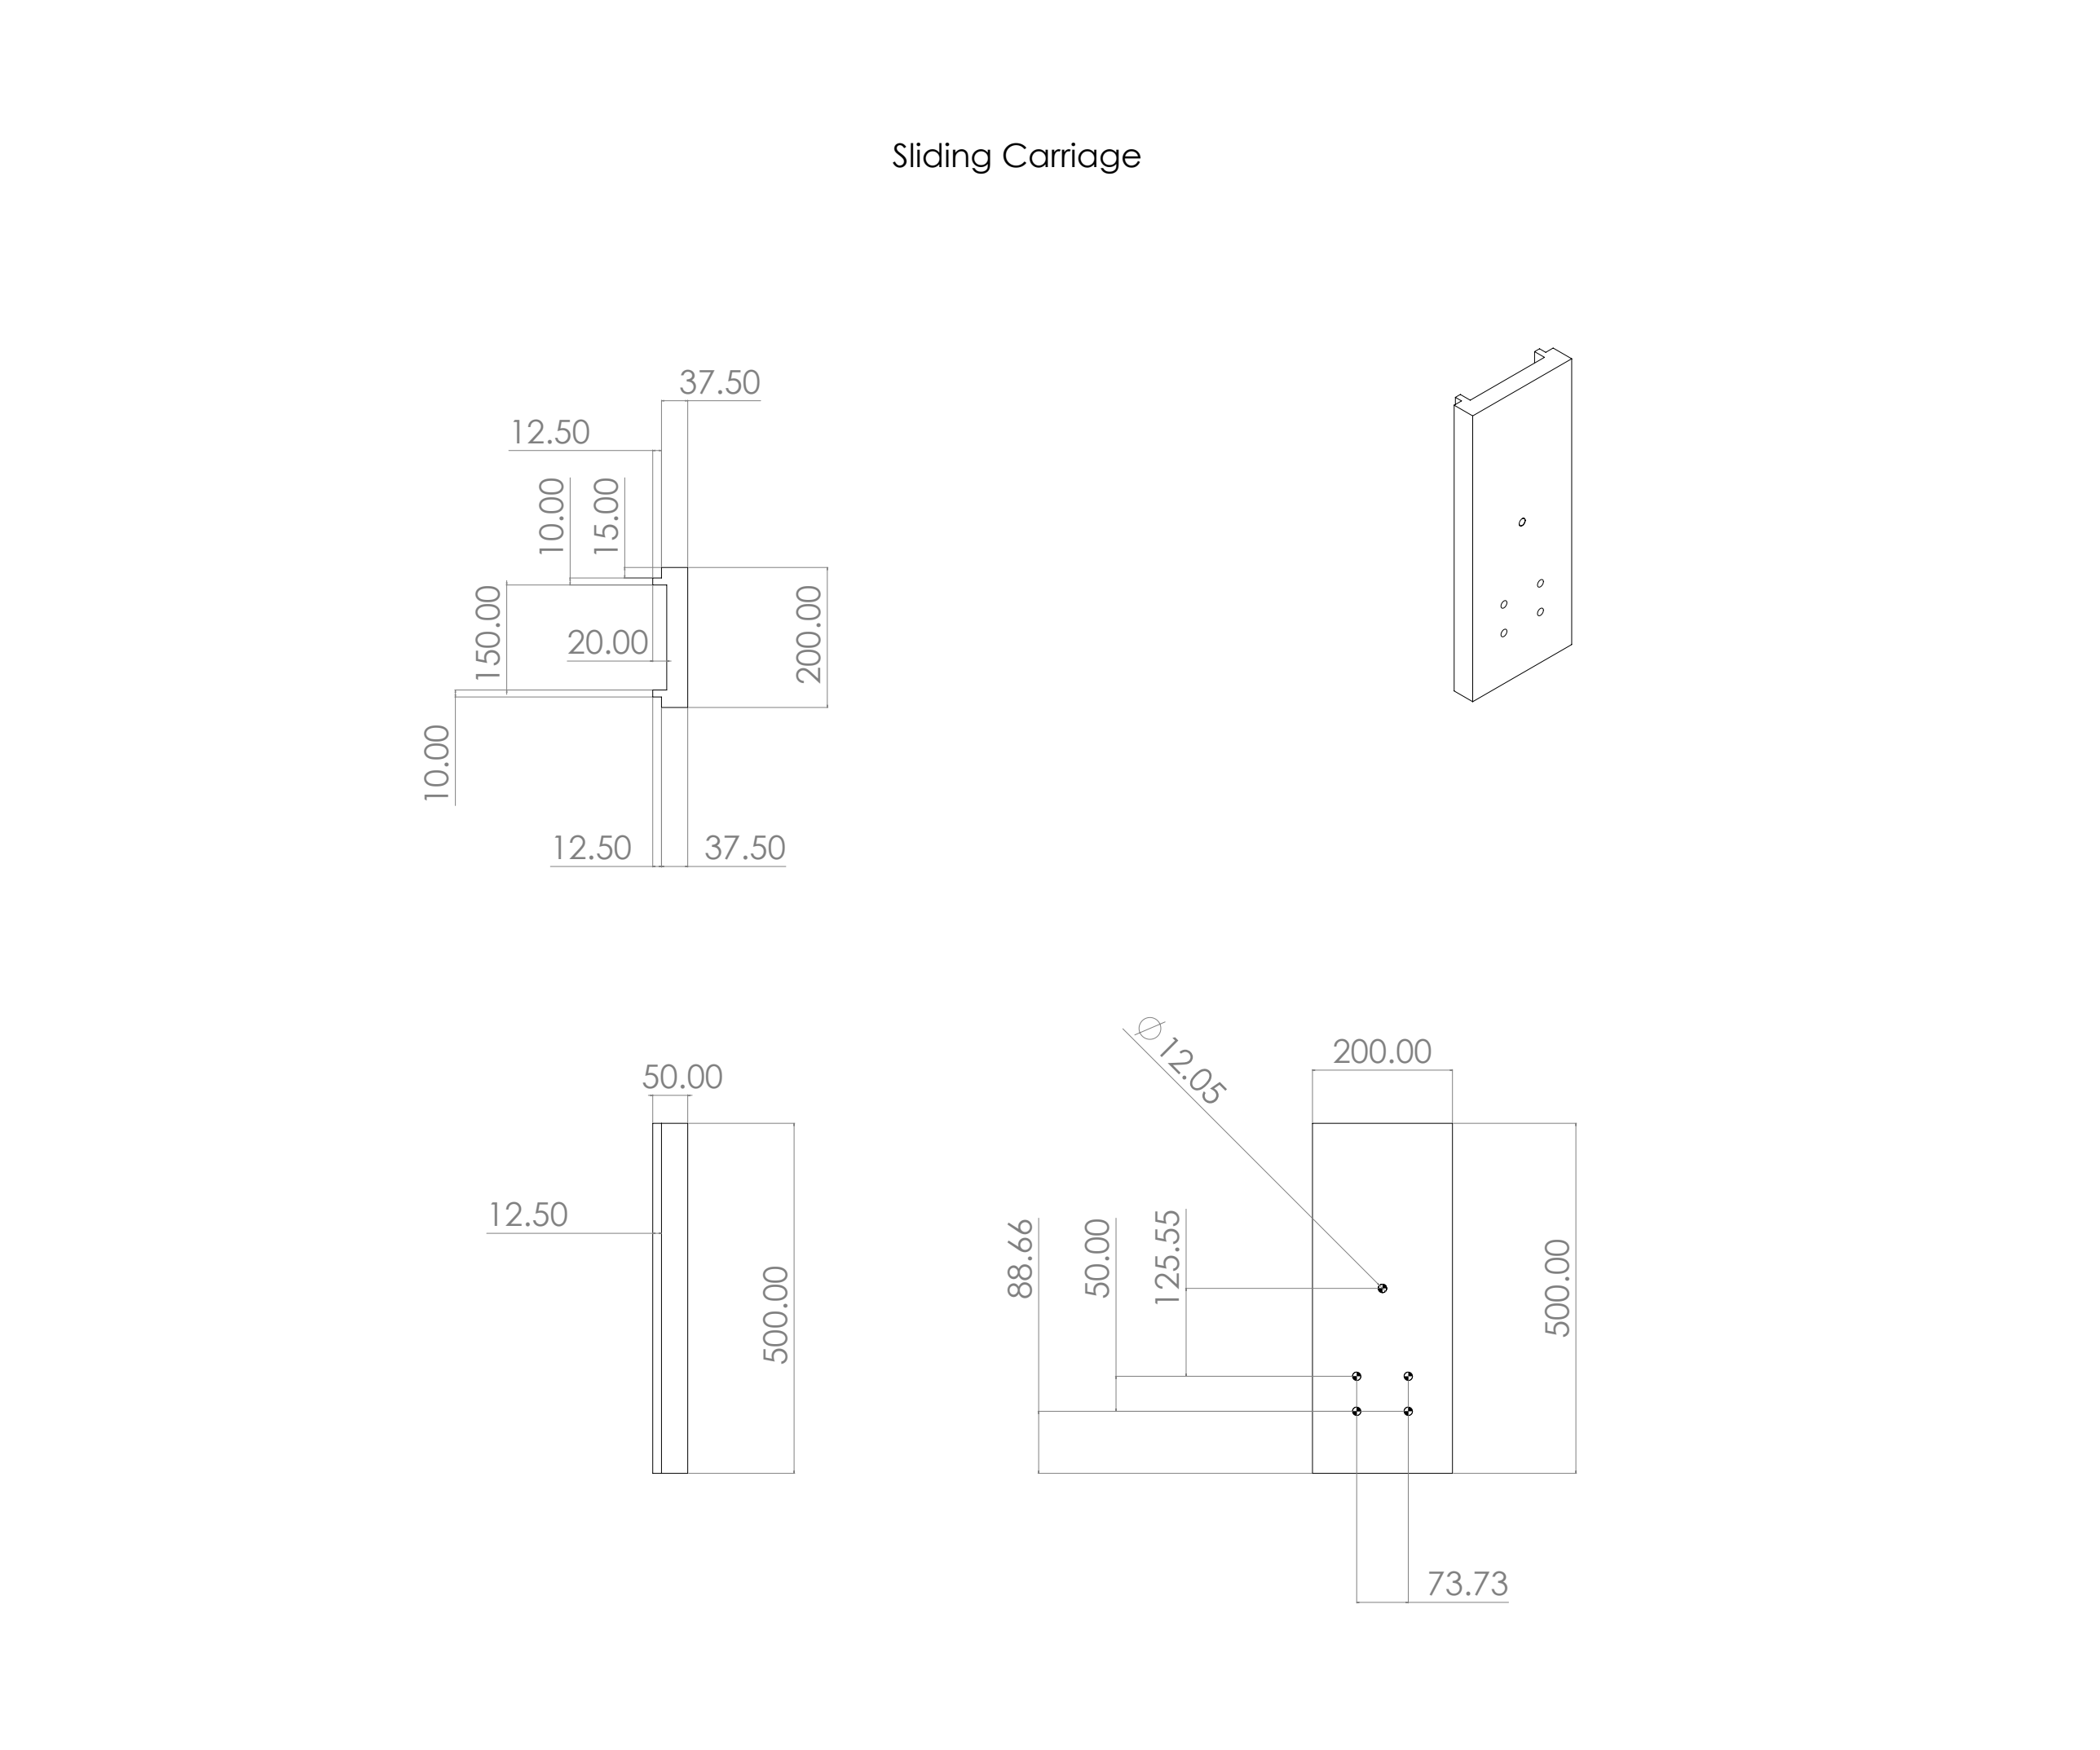
ISO-10303-21;
HEADER;
FILE_DESCRIPTION (('STEP AP214'),
    '1' );
FILE_NAME ('Sliding Carriage.step',
    '2026-10-24T00:09:50',
    ( '' ),
    ( '' ),
    'SwSTEP 2.0',
    'SolidWorks 2025',
    '' );
FILE_SCHEMA (( 'AUTOMOTIVE_DESIGN' ));
ENDSEC;

DATA;
#23=DIRECTION ( 'NONE',  ( 0.000000000000000000, 0.000000000000000000, -1.000000000000000000 ) ) ;
#76=EDGE_LOOP ( 'NONE', ( #23237, #5440, #9626, #3047 ) ) ;
#80=DIRECTION ( 'NONE',  ( 0.000000000000000000, 0.000000000000000000, -1.000000000000000000 ) ) ;
#130=CARTESIAN_POINT ( 'NONE',  ( 217.4999999999996305, -5.589247009368136787, -100.0000000000000142 ) ) ;
#156=DIRECTION ( 'NONE',  ( 0.000000000000000000, 0.000000000000000000, -1.000000000000000000 ) ) ;
#159=AXIS2_PLACEMENT_3D ( 'NONE', #7876, #3416, #12207 ) ;
#181=CARTESIAN_POINT ( 'NONE',  ( 217.4999999999996305, 133.0668745871126930, -36.86484227207694886 ) ) ;
#186=PRODUCT_DEFINITION ( 'UNKNOWN', '', #23049, #8609 ) ;
#209=DIRECTION ( 'NONE',  ( 0.000000000000000000, 0.000000000000000000, -1.000000000000000000 ) ) ;
#238=ADVANCED_FACE ( 'NONE', ( #10870 ), #21904, .F. ) ;
#434=ORIENTED_EDGE ( 'NONE', *, *, #7614, .T. ) ;
#444=ORIENTED_EDGE ( 'NONE', *, *, #19204, .F. ) ;
#447=EDGE_LOOP ( 'NONE', ( #17565, #15243, #25837, #22811 ) ) ;
#472=ADVANCED_FACE ( 'NONE', ( #8071 ), #26010, .F. ) ;
#488=DIRECTION ( 'NONE',  ( 1.000000000000000000, -0.000000000000000000, 0.000000000000000000 ) ) ;
#531=CARTESIAN_POINT ( 'NONE',  ( 167.4999999999996589, -5.589247009368137675, -74.99999999999995737 ) ) ;
#607=CARTESIAN_POINT ( 'NONE',  ( 217.4999999999996305, 133.0668745871126930, 36.86484227207694886 ) ) ;
#610=CARTESIAN_POINT ( 'NONE',  ( 187.4999999999996305, 258.6181251126050711, 1.387778780781445676E-14 ) ) ;
#662=DIRECTION ( 'NONE',  ( 0.000000000000000000, 1.214306433183764966E-16, -1.000000000000000000 ) ) ;
#674=EDGE_CURVE ( 'NONE', #21518, #27627, #20135, .T. ) ;
#676=FACE_OUTER_BOUND ( 'NONE', #18606, .T. ) ;
#754=ORIENTED_EDGE ( 'NONE', *, *, #21243, .F. ) ;
#812=LINE ( 'NONE', #948, #4384 ) ;
#831=EDGE_CURVE ( 'NONE', #3911, #16933, #25279, .T. ) ;
#948=CARTESIAN_POINT ( 'NONE',  ( 187.4999999999996305, 526.4263741777961059, -74.99999999999995737 ) ) ;
#968=VERTEX_POINT ( 'NONE', #19378 ) ;
#1018=EDGE_CURVE ( 'NONE', #9020, #6014, #12368, .T. ) ;
#1093=ORIENTED_EDGE ( 'NONE', *, *, #14518, .F. ) ;
#1099=( NAMED_UNIT ( * ) PLANE_ANGLE_UNIT ( ) SI_UNIT ( $, .RADIAN. ) );
#1105=DIRECTION ( 'NONE',  ( 0.000000000000000000, 0.000000000000000000, -1.000000000000000000 ) ) ;
#1147=DIRECTION ( 'NONE',  ( -0.000000000000000000, -1.000000000000000000, -0.000000000000000000 ) ) ;
#1186=FACE_OUTER_BOUND ( 'NONE', #26674, .T. ) ;
#1194=FACE_OUTER_BOUND ( 'NONE', #5435, .T. ) ;
#1240=CARTESIAN_POINT ( 'NONE',  ( 167.4999999999996589, 494.4107529906318632, -74.99999999999995737 ) ) ;
#1265=CARTESIAN_POINT ( 'NONE',  ( 167.4999999999996589, 526.4263741777961059, 74.99999999999995737 ) ) ;
#1291=FACE_BOUND ( 'NONE', #15259, .T. ) ;
#1308=EDGE_CURVE ( 'NONE', #19372, #18272, #13460, .T. ) ;
#1373=EDGE_CURVE ( 'NONE', #24637, #27485, #4396, .T. ) ;
#1377=ORIENTED_EDGE ( 'NONE', *, *, #15555, .T. ) ;
#1470=CARTESIAN_POINT ( 'NONE',  ( 179.9999999999999147, 526.4263741777961059, 84.99999999999997158 ) ) ;
#1516=CARTESIAN_POINT ( 'NONE',  ( 232.4999999999996305, 133.0668745871126930, -36.86484227207694886 ) ) ;
#1540=EDGE_CURVE ( 'NONE', #2445, #22920, #20876, .T. ) ;
#1543=DIRECTION ( 'NONE',  ( 1.000000000000000000, 0.000000000000000000, 0.000000000000000000 ) ) ;
#1687=FACE_BOUND ( 'NONE', #7272, .T. ) ;
#1713=CARTESIAN_POINT ( 'NONE',  ( 187.4999999999996305, 133.0668745871126930, 30.86484227207697018 ) ) ;
#1717=DIRECTION ( 'NONE',  ( -1.000000000000000000, -0.000000000000000000, -0.000000000000000000 ) ) ;
#1723=LINE ( 'NONE', #23710, #21354 ) ;
#1774=DIRECTION ( 'NONE',  ( 1.000000000000000000, 0.000000000000000000, 0.000000000000000000 ) ) ;
#1831=ORIENTED_EDGE ( 'NONE', *, *, #2595, .F. ) ;
#1859=AXIS2_PLACEMENT_3D ( 'NONE', #1470, #21003, #18999 ) ;
#1932=CIRCLE ( 'NONE', #12073, 6.025000000000002132 ) ;
#1988=VECTOR ( 'NONE', #19866, 1000.000000000000000 ) ;
#1994=LINE ( 'NONE', #4004, #23887 ) ;
#2014=ORIENTED_EDGE ( 'NONE', *, *, #1373, .T. ) ;
#2128=AXIS2_PLACEMENT_3D ( 'NONE', #17004, #16870, #21173 ) ;
#2140=EDGE_CURVE ( 'NONE', #14281, #9708, #7935, .T. ) ;
#2141=DIRECTION ( 'NONE',  ( 1.000000000000000000, -0.000000000000000000, -0.000000000000000000 ) ) ;
#2152=ORIENTED_EDGE ( 'NONE', *, *, #23804, .T. ) ;
#2172=ADVANCED_FACE ( 'NONE', ( #1186 ), #23024, .F. ) ;
#2183=DIRECTION ( 'NONE',  ( 1.000000000000000000, -0.000000000000000000, -0.000000000000000000 ) ) ;
#2195=FACE_OUTER_BOUND ( 'NONE', #8358, .T. ) ;
#2207=ORIENTED_EDGE ( 'NONE', *, *, #674, .F. ) ;
#2214=LINE ( 'NONE', #11000, #23023 ) ;
#2291=DIRECTION ( 'NONE',  ( 1.000000000000000000, 0.000000000000000000, 0.000000000000000000 ) ) ;
#2302=CARTESIAN_POINT ( 'NONE',  ( 232.4999999999996305, 83.06687458711267880, -36.86484227207694175 ) ) ;
#2303=LINE ( 'NONE', #9071, #27272 ) ;
#2320=DIRECTION ( 'NONE',  ( 0.000000000000000000, 0.000000000000000000, 1.000000000000000000 ) ) ;
#2328=DIRECTION ( 'NONE',  ( 1.000000000000000000, 0.000000000000000000, 0.000000000000000000 ) ) ;
#2330=LINE ( 'NONE', #11110, #4291 ) ;
#2345=CARTESIAN_POINT ( 'NONE',  ( 217.4999999999996305, -5.589247009368136787, -100.0000000000000142 ) ) ;
#2445=VERTEX_POINT ( 'NONE', #23522 ) ;
#2509=ORIENTED_EDGE ( 'NONE', *, *, #18393, .F. ) ;
#2560=DIRECTION ( 'NONE',  ( 1.000000000000000000, 0.000000000000000000, -0.000000000000000000 ) ) ;
#2595=EDGE_CURVE ( 'NONE', #16577, #4345, #812, .T. ) ;
#2599=EDGE_CURVE ( 'NONE', #26389, #3911, #9715, .T. ) ;
#2677=AXIS2_PLACEMENT_3D ( 'NONE', #19216, #27958, #8304 ) ;
#2691=VECTOR ( 'NONE', #2141, 1000.000000000000000 ) ;
#2703=AXIS2_PLACEMENT_3D ( 'NONE', #17117, #10232, #25727 ) ;
#2750=ADVANCED_FACE ( 'NONE', ( #676 ), #18614, .F. ) ;
#2774=CARTESIAN_POINT ( 'NONE',  ( 179.9999999999999147, 494.4107529906318632, 84.99999999999997158 ) ) ;
#2821=VECTOR ( 'NONE', #7715, 1000.000000000000000 ) ;
#2843=ADVANCED_FACE ( 'NONE', ( #27915 ), #23630, .F. ) ;
#2855=VECTOR ( 'NONE', #24756, 1000.000000000000114 ) ;
#2867=CARTESIAN_POINT ( 'NONE',  ( 217.4999999999996305, 258.6181251126050711, 1.387778780781445676E-14 ) ) ;
#2909=ORIENTED_EDGE ( 'NONE', *, *, #14447, .T. ) ;
#2932=ORIENTED_EDGE ( 'NONE', *, *, #18092, .T. ) ;
#2962=AXIS2_PLACEMENT_3D ( 'NONE', #11758, #16063, #7143 ) ;
#3012=VERTEX_POINT ( 'NONE', #4639 ) ;
#3018=CARTESIAN_POINT ( 'NONE',  ( 179.9999999999999147, 526.4263741777961059, 84.99999999999997158 ) ) ;
#3039=DIRECTION ( 'NONE',  ( 0.000000000000000000, 0.000000000000000000, -1.000000000000000000 ) ) ;
#3047=ORIENTED_EDGE ( 'NONE', *, *, #13106, .T. ) ;
#3137=AXIS2_PLACEMENT_3D ( 'NONE', #1516, #23639, #8272 ) ;
#3294=CARTESIAN_POINT ( 'NONE',  ( 217.4999999999996305, 133.0668745871126930, -42.86484227207692044 ) ) ;
#3375=DIRECTION ( 'NONE',  ( -0.000000000000000000, -1.000000000000000000, -0.000000000000000000 ) ) ;
#3393=ORIENTED_EDGE ( 'NONE', *, *, #12066, .T. ) ;
#3416=DIRECTION ( 'NONE',  ( 1.000000000000000000, -0.000000000000000000, -0.000000000000000000 ) ) ;
#3440=FACE_OUTER_BOUND ( 'NONE', #12942, .T. ) ;
#3482=PLANE ( 'NONE',  #1859 ) ;
#3485=DIRECTION ( 'NONE',  ( -0.000000000000000000, -1.000000000000000000, -0.000000000000000000 ) ) ;
#3548=EDGE_CURVE ( 'NONE', #14563, #14477, #8151, .T. ) ;
#3578=APPLICATION_CONTEXT ( 'automotive_design' ) ;
#3643=CARTESIAN_POINT ( 'NONE',  ( 179.9999999999999147, 494.4107529906318632, -84.99999999999997158 ) ) ;
#3655=DIRECTION ( 'NONE',  ( 0.000000000000000000, 1.214306433183764966E-16, -1.000000000000000000 ) ) ;
#3669=CARTESIAN_POINT ( 'NONE',  ( 217.4999999999996305, 258.6181251126050711, -6.024999999999988809 ) ) ;
#3670=ORIENTED_EDGE ( 'NONE', *, *, #19154, .F. ) ;
#3672=CARTESIAN_POINT ( 'NONE',  ( 187.4999999999996305, 83.06687458711267880, 36.86484227207694175 ) ) ;
#3718=PLANE ( 'NONE',  #15616 ) ;
#3764=DIRECTION ( 'NONE',  ( 0.000000000000000000, 0.000000000000000000, -1.000000000000000000 ) ) ;
#3773=DIRECTION ( 'NONE',  ( 1.000000000000000000, 0.000000000000000000, 0.000000000000000000 ) ) ;
#3791=VECTOR ( 'NONE', #9849, 1000.000000000000000 ) ;
#3793=VECTOR ( 'NONE', #15027, 1000.000000000000000 ) ;
#3831=AXIS2_PLACEMENT_3D ( 'NONE', #4036, #23304, #14688 ) ;
#3866=VECTOR ( 'NONE', #13181, 1000.000000000000000 ) ;
#3911=VERTEX_POINT ( 'NONE', #2774 ) ;
#3960=VECTOR ( 'NONE', #8586, 1000.000000000000000 ) ;
#3996=CLOSED_SHELL ( 'NONE', ( #238, #10166, #22536, #16043, #17421, #2843, #6982, #24610, #18673, #17163, #2172, #4904, #27874, #18220, #23426, #4744, #19820, #15702, #472, #22099, #11379, #22428, #2750, #12885, #26047, #15496 ) ) ;
#4004=CARTESIAN_POINT ( 'NONE',  ( 232.4999999999996305, 83.06687458711267880, 42.86484227207692754 ) ) ;
#4036=CARTESIAN_POINT ( 'NONE',  ( 232.4999999999996305, 133.0668745871126930, 36.86484227207694886 ) ) ;
#4092=CARTESIAN_POINT ( 'NONE',  ( 167.4999999999996589, 494.4107529906318632, 84.99999999999995737 ) ) ;
#4145=CARTESIAN_POINT ( 'NONE',  ( 167.4999999999996589, 526.4263741777961059, 84.99999999999995737 ) ) ;
#4184=DIRECTION ( 'NONE',  ( -0.000000000000000000, -1.000000000000000000, -0.000000000000000000 ) ) ;
#4242=EDGE_LOOP ( 'NONE', ( #26927, #2909, #13178, #28392 ) ) ;
#4270=CARTESIAN_POINT ( 'NONE',  ( 179.9999999999999147, 526.4263741777961059, -100.0000000000000142 ) ) ;
#4291=VECTOR ( 'NONE', #4351, 1000.000000000000000 ) ;
#4345=VERTEX_POINT ( 'NONE', #16950 ) ;
#4351=DIRECTION ( 'NONE',  ( -0.000000000000000000, -1.000000000000000000, -0.000000000000000000 ) ) ;
#4377=EDGE_LOOP ( 'NONE', ( #16558, #1093 ) ) ;
#4384=VECTOR ( 'NONE', #3375, 1000.000000000000000 ) ;
#4396=LINE ( 'NONE', #24224, #25465 ) ;
#4419=ORIENTED_EDGE ( 'NONE', *, *, #26008, .F. ) ;
#4443=ORIENTED_EDGE ( 'NONE', *, *, #17601, .F. ) ;
#4499=CARTESIAN_POINT ( 'NONE',  ( 217.4999999999996305, 83.06687458711267880, 36.86484227207694175 ) ) ;
#4524=ORIENTED_EDGE ( 'NONE', *, *, #10490, .T. ) ;
#4529=DIRECTION ( 'NONE',  ( 0.000000000000000000, 1.214306433183764966E-16, -1.000000000000000000 ) ) ;
#4541=FACE_BOUND ( 'NONE', #24827, .T. ) ;
#4545=VECTOR ( 'NONE', #1147, 1000.000000000000000 ) ;
#4562=VERTEX_POINT ( 'NONE', #22830 ) ;
#4581=LINE ( 'NONE', #11062, #27172 ) ;
#4624=EDGE_CURVE ( 'NONE', #9708, #968, #5408, .T. ) ;
#4639=CARTESIAN_POINT ( 'NONE',  ( 187.4999999999996305, 83.06687458711267880, 42.86484227207692754 ) ) ;
#4641=DIRECTION ( 'NONE',  ( 0.000000000000000000, 1.214306433183764966E-16, -1.000000000000000000 ) ) ;
#4660=CARTESIAN_POINT ( 'NONE',  ( 217.4749999999996533, 258.6181251126050711, 1.387778780781445676E-14 ) ) ;
#4661=VERTEX_POINT ( 'NONE', #14494 ) ;
#4676=VECTOR ( 'NONE', #19046, 1000.000000000000114 ) ;
#4730=DIRECTION ( 'NONE',  ( 0.000000000000000000, 0.000000000000000000, -1.000000000000000000 ) ) ;
#4744=ADVANCED_FACE ( 'NONE', ( #14351 ), #20810, .F. ) ;
#4763=DIRECTION ( 'NONE',  ( 0.000000000000000000, 0.000000000000000000, -1.000000000000000000 ) ) ;
#4766=SHAPE_REPRESENTATION_RELATIONSHIP ( 'NONE' , 'NONE' ,  #13220, #16401 ) ;
#4871=ORIENTED_EDGE ( 'NONE', *, *, #15555, .F. ) ;
#4904=ADVANCED_FACE ( 'NONE', ( #24232, #15346, #4541, #13329, #1687, #17202 ), #10455, .T. ) ;
#4932=DIRECTION ( 'NONE',  ( 0.000000000000000000, 0.000000000000000000, -1.000000000000000000 ) ) ;
#4964=DIRECTION ( 'NONE',  ( 1.000000000000000000, 0.000000000000000000, -2.220446049250266932E-15 ) ) ;
#5041=DIRECTION ( 'NONE',  ( 1.000000000000000000, 0.000000000000000000, 0.000000000000000000 ) ) ;
#5050=( LENGTH_UNIT ( ) NAMED_UNIT ( * ) SI_UNIT ( .MILLI., .METRE. ) );
#5100=CARTESIAN_POINT ( 'NONE',  ( 179.9999999999999147, -5.589247009368164321, 100.0000000000000142 ) ) ;
#5115=CARTESIAN_POINT ( 'NONE',  ( 217.4999999999996305, -5.589247009368136787, -100.0000000000000142 ) ) ;
#5154=DIRECTION ( 'NONE',  ( 1.000000000000000000, 0.000000000000000000, 0.000000000000000000 ) ) ;
#5161=VECTOR ( 'NONE', #4964, 1000.000000000000000 ) ;
#5228=ORIENTED_EDGE ( 'NONE', *, *, #21351, .T. ) ;
#5234=EDGE_LOOP ( 'NONE', ( #27799, #10042 ) ) ;
#5314=VECTOR ( 'NONE', #8613, 1000.000000000000000 ) ;
#5360=LINE ( 'NONE', #27193, #24321 ) ;
#5408=CIRCLE ( 'NONE', #12320, 5.999999999999991118 ) ;
#5412=AXIS2_PLACEMENT_3D ( 'NONE', #6491, #22144, #17691 ) ;
#5435=EDGE_LOOP ( 'NONE', ( #22782, #8591, #26320, #25041 ) ) ;
#5437=LINE ( 'NONE', #26991, #17052 ) ;
#5440=ORIENTED_EDGE ( 'NONE', *, *, #20755, .F. ) ;
#5552=VECTOR ( 'NONE', #1717, 1000.000000000000000 ) ;
#5601=FACE_BOUND ( 'NONE', #12836, .T. ) ;
#5612=DIRECTION ( 'NONE',  ( 0.000000000000000000, 0.000000000000000000, -1.000000000000000000 ) ) ;
#5630=CIRCLE ( 'NONE', #14831, 6.000000000000005329 ) ;
#5696=CARTESIAN_POINT ( 'NONE',  ( 167.4999999999996589, -5.589247009368157215, 84.99999999999995737 ) ) ;
#5733=ORIENTED_EDGE ( 'NONE', *, *, #20344, .F. ) ;
#5740=FACE_BOUND ( 'NONE', #5234, .T. ) ;
#5863=ORIENTED_EDGE ( 'NONE', *, *, #7192, .F. ) ;
#5876=VECTOR ( 'NONE', #4641, 1000.000000000000000 ) ;
#5889=DIRECTION ( 'NONE',  ( -1.000000000000000000, 0.000000000000000000, -0.000000000000000000 ) ) ;
#5958=DIRECTION ( 'NONE',  ( 0.000000000000000000, 0.000000000000000000, -1.000000000000000000 ) ) ;
#5977=EDGE_LOOP ( 'NONE', ( #22241, #22737, #9263, #8482 ) ) ;
#6014=VERTEX_POINT ( 'NONE', #8020 ) ;
#6087=FACE_OUTER_BOUND ( 'NONE', #26011, .T. ) ;
#6120=CIRCLE ( 'NONE', #24934, 5.999999999999977796 ) ;
#6124=EDGE_LOOP ( 'NONE', ( #8360, #14998 ) ) ;
#6204=LINE ( 'NONE', #9481, #25732 ) ;
#6337=EDGE_CURVE ( 'NONE', #3012, #14281, #16973, .T. ) ;
#6488=VECTOR ( 'NONE', #17209, 1000.000000000000000 ) ;
#6491=CARTESIAN_POINT ( 'NONE',  ( 187.4999999999996305, 133.0668745871126930, 36.86484227207694886 ) ) ;
#6510=DIRECTION ( 'NONE',  ( 0.000000000000000000, 0.000000000000000000, -1.000000000000000000 ) ) ;
#6525=AXIS2_PLACEMENT_3D ( 'NONE', #610, #13832, #22998 ) ;
#6568=LINE ( 'NONE', #13467, #10167 ) ;
#6644=AXIS2_PLACEMENT_3D ( 'NONE', #12015, #20759, #26808 ) ;
#6671=DIRECTION ( 'NONE',  ( 1.000000000000000000, 0.000000000000000000, 0.000000000000000000 ) ) ;
#6681=CARTESIAN_POINT ( 'NONE',  ( 232.4999999999996305, 133.0668745871126930, -30.86484227207697018 ) ) ;
#6723=CIRCLE ( 'NONE', #15462, 5.999999999999991118 ) ;
#6776=CIRCLE ( 'NONE', #5412, 5.999999999999977796 ) ;
#6861=( GEOMETRIC_REPRESENTATION_CONTEXT ( 3 ) GLOBAL_UNCERTAINTY_ASSIGNED_CONTEXT ( ( #8892 ) ) GLOBAL_UNIT_ASSIGNED_CONTEXT ( ( #10431, #1099, #18624 ) ) REPRESENTATION_CONTEXT ( 'NONE', 'WORKASPACE' ) );
#6878=CIRCLE ( 'NONE', #21556, 6.000000000000005329 ) ;
#6907=DIRECTION ( 'NONE',  ( 1.000000000000000000, -0.000000000000000000, -0.000000000000000000 ) ) ;
#6935=ORIENTED_EDGE ( 'NONE', *, *, #15210, .F. ) ;
#6982=ADVANCED_FACE ( 'NONE', ( #7898, #1291, #5601, #12089, #5740, #3440 ), #3718, .F. ) ;
#7037=VERTEX_POINT ( 'NONE', #18815 ) ;
#7044=VERTEX_POINT ( 'NONE', #3294 ) ;
#7143=DIRECTION ( 'NONE',  ( 0.000000000000000000, 0.000000000000000000, -1.000000000000000000 ) ) ;
#7192=EDGE_CURVE ( 'NONE', #3012, #968, #1994, .T. ) ;
#7229=CARTESIAN_POINT ( 'NONE',  ( 179.9999999999999147, 494.4107529906318632, 100.0000000000000142 ) ) ;
#7272=EDGE_LOOP ( 'NONE', ( #15212, #22647 ) ) ;
#7306=CARTESIAN_POINT ( 'NONE',  ( 217.4999999999996305, 258.6181251126050711, -6.024999999999988809 ) ) ;
#7316=EDGE_CURVE ( 'NONE', #6014, #27664, #26379, .T. ) ;
#7374=ORIENTED_EDGE ( 'NONE', *, *, #19154, .T. ) ;
#7422=VECTOR ( 'NONE', #18205, 1000.000000000000000 ) ;
#7439=DIRECTION ( 'NONE',  ( 1.000000000000000000, -0.000000000000000000, 0.000000000000000000 ) ) ;
#7614=EDGE_CURVE ( 'NONE', #4345, #24637, #24167, .T. ) ;
#7615=LINE ( 'NONE', #10045, #10208 ) ;
#7654=CARTESIAN_POINT ( 'NONE',  ( 217.4999999999996305, 258.6181251126050711, 6.025000000000016342 ) ) ;
#7689=ORIENTED_EDGE ( 'NONE', *, *, #10328, .T. ) ;
#7715=DIRECTION ( 'NONE',  ( -1.000000000000000000, 0.000000000000000000, 0.000000000000000000 ) ) ;
#7761=AXIS2_PLACEMENT_3D ( 'NONE', #20264, #26876, #11372 ) ;
#7806=DIRECTION ( 'NONE',  ( 1.000000000000000000, -0.000000000000000000, -0.000000000000000000 ) ) ;
#7876=CARTESIAN_POINT ( 'NONE',  ( 232.4999999999996305, 83.06687458711267880, 36.86484227207694175 ) ) ;
#7887=( GEOMETRIC_REPRESENTATION_CONTEXT ( 3 ) GLOBAL_UNCERTAINTY_ASSIGNED_CONTEXT ( ( #15510 ) ) GLOBAL_UNIT_ASSIGNED_CONTEXT ( ( #5050, #13550, #11249 ) ) REPRESENTATION_CONTEXT ( 'NONE', 'WORKASPACE' ) );
#7898=FACE_BOUND ( 'NONE', #6124, .T. ) ;
#7935=LINE ( 'NONE', #18710, #5314 ) ;
#7944=LINE ( 'NONE', #23174, #27418 ) ;
#7965=ORIENTED_EDGE ( 'NONE', *, *, #21218, .T. ) ;
#7994=EDGE_CURVE ( 'NONE', #13277, #27664, #21545, .T. ) ;
#8020=CARTESIAN_POINT ( 'NONE',  ( 179.9999999999999147, 494.4107529906318632, -100.0000000000000142 ) ) ;
#8030=VERTEX_POINT ( 'NONE', #9339 ) ;
#8050=CARTESIAN_POINT ( 'NONE',  ( 167.4999999999996589, 526.4263741777961059, -74.99999999999995737 ) ) ;
#8066=VERTEX_POINT ( 'NONE', #26415 ) ;
#8071=FACE_OUTER_BOUND ( 'NONE', #19006, .T. ) ;
#8081=CARTESIAN_POINT ( 'NONE',  ( 217.4999999999996305, 83.06687458711267880, -30.86484227207694886 ) ) ;
#8120=EDGE_CURVE ( 'NONE', #4661, #21276, #9706, .T. ) ;
#8151=LINE ( 'NONE', #27672, #23338 ) ;
#8247=CYLINDRICAL_SURFACE ( 'NONE', #2128, 6.000000000000005329 ) ;
#8251=EDGE_CURVE ( 'NONE', #16577, #24145, #5437, .T. ) ;
#8263=CARTESIAN_POINT ( 'NONE',  ( 232.4999999999996305, 83.06687458711267880, 36.86484227207694175 ) ) ;
#8272=DIRECTION ( 'NONE',  ( 0.000000000000000000, 0.000000000000000000, -1.000000000000000000 ) ) ;
#8300=EDGE_CURVE ( 'NONE', #22920, #7044, #12772, .T. ) ;
#8304=DIRECTION ( 'NONE',  ( 0.000000000000000000, 0.000000000000000000, -1.000000000000000000 ) ) ;
#8351=EDGE_LOOP ( 'NONE', ( #13470, #21698, #13841, #10543 ) ) ;
#8358=EDGE_LOOP ( 'NONE', ( #19886, #23578, #13452, #14559 ) ) ;
#8360=ORIENTED_EDGE ( 'NONE', *, *, #17601, .T. ) ;
#8412=CYLINDRICAL_SURFACE ( 'NONE', #3137, 5.999999999999977796 ) ;
#8415=CARTESIAN_POINT ( 'NONE',  ( 187.4999999999996305, 133.0668745871126930, 42.86484227207692044 ) ) ;
#8482=ORIENTED_EDGE ( 'NONE', *, *, #26274, .T. ) ;
#8511=EDGE_LOOP ( 'NONE', ( #20997, #1377 ) ) ;
#8552=CARTESIAN_POINT ( 'NONE',  ( 217.4999999999996305, -5.589247009368160768, 100.0000000000000142 ) ) ;
#8578=EDGE_CURVE ( 'NONE', #16577, #18911, #22939, .T. ) ;
#8586=DIRECTION ( 'NONE',  ( 1.000000000000000000, -0.000000000000000000, -0.000000000000000000 ) ) ;
#8591=ORIENTED_EDGE ( 'NONE', *, *, #9752, .F. ) ;
#8609=PRODUCT_DEFINITION_CONTEXT ( 'detailed design', #10391, 'design' ) ;
#8613=DIRECTION ( 'NONE',  ( 1.000000000000000000, -0.000000000000000000, -0.000000000000000000 ) ) ;
#8650=VERTEX_POINT ( 'NONE', #5696 ) ;
#8726=ORIENTED_EDGE ( 'NONE', *, *, #1540, .T. ) ;
#8742=EDGE_CURVE ( 'NONE', #21276, #21518, #23357, .T. ) ;
#8810=ORIENTED_EDGE ( 'NONE', *, *, #10328, .F. ) ;
#8845=EDGE_CURVE ( 'NONE', #2445, #17060, #17452, .T. ) ;
#8847=EDGE_CURVE ( 'NONE', #20391, #27472, #2214, .T. ) ;
#8881=EDGE_LOOP ( 'NONE', ( #14167, #5228, #21092, #21123 ) ) ;
#8892=UNCERTAINTY_MEASURE_WITH_UNIT (LENGTH_MEASURE( 1.000000000000000082E-05 ), #10431, 'distance_accuracy_value', 'NONE');
#8984=DIRECTION ( 'NONE',  ( 1.000000000000000000, -0.000000000000000000, -0.000000000000000000 ) ) ;
#8993=CARTESIAN_POINT ( 'NONE',  ( 179.9999999999999147, 494.4107529906318632, -100.0000000000000142 ) ) ;
#9020=VERTEX_POINT ( 'NONE', #14997 ) ;
#9035=DIRECTION ( 'NONE',  ( -1.000000000000000000, -0.000000000000000000, -0.000000000000000000 ) ) ;
#9040=DIRECTION ( 'NONE',  ( 0.000000000000000000, -1.214306433183764966E-16, 1.000000000000000000 ) ) ;
#9052=CARTESIAN_POINT ( 'NONE',  ( 187.4999999999996305, -5.589247009368136787, -100.0000000000000142 ) ) ;
#9058=CARTESIAN_POINT ( 'NONE',  ( 187.4999999999996305, 83.06687458711267880, -36.86484227207694175 ) ) ;
#9071=CARTESIAN_POINT ( 'NONE',  ( 179.9999999999999147, 494.4107529906318632, 84.99999999999997158 ) ) ;
#9075=DIRECTION ( 'NONE',  ( 0.000000000000000000, 0.000000000000000000, -1.000000000000000000 ) ) ;
#9170=ORIENTED_EDGE ( 'NONE', *, *, #9262, .T. ) ;
#9177=EDGE_CURVE ( 'NONE', #27627, #21518, #1932, .T. ) ;
#9235=FACE_OUTER_BOUND ( 'NONE', #8351, .T. ) ;
#9262=EDGE_CURVE ( 'NONE', #25171, #22044, #7615, .T. ) ;
#9263=ORIENTED_EDGE ( 'NONE', *, *, #19204, .T. ) ;
#9330=LINE ( 'NONE', #13081, #25969 ) ;
#9339=CARTESIAN_POINT ( 'NONE',  ( 187.4999999999996305, 258.6181251126050711, 6.000000000000019540 ) ) ;
#9349=VECTOR ( 'NONE', #17501, 1000.000000000000000 ) ;
#9355=CIRCLE ( 'NONE', #14396, 5.999999999999977796 ) ;
#9393=CARTESIAN_POINT ( 'NONE',  ( 167.4999999999996589, -5.589247009368136787, -84.99999999999995737 ) ) ;
#9418=LINE ( 'NONE', #20606, #26682 ) ;
#9442=LINE ( 'NONE', #15913, #5161 ) ;
#9445=LINE ( 'NONE', #27363, #7422 ) ;
#9448=ORIENTED_EDGE ( 'NONE', *, *, #8578, .F. ) ;
#9464=EDGE_LOOP ( 'NONE', ( #2509, #21032, #20003, #24207 ) ) ;
#9481=CARTESIAN_POINT ( 'NONE',  ( 167.4999999999996589, 526.4263741777961059, -74.99999999999995737 ) ) ;
#9533=CARTESIAN_POINT ( 'NONE',  ( 217.4999999999996305, 133.0668745871126930, 42.86484227207692044 ) ) ;
#9596=ORIENTED_EDGE ( 'NONE', *, *, #14518, .T. ) ;
#9626=ORIENTED_EDGE ( 'NONE', *, *, #15888, .T. ) ;
#9683=EDGE_CURVE ( 'NONE', #14281, #3012, #18431, .T. ) ;
#9690=ORIENTED_EDGE ( 'NONE', *, *, #7994, .F. ) ;
#9706=CIRCLE ( 'NONE', #13376, 6.000000000000005329 ) ;
#9708=VERTEX_POINT ( 'NONE', #14897 ) ;
#9715=LINE ( 'NONE', #27090, #21369 ) ;
#9752=EDGE_CURVE ( 'NONE', #21276, #4661, #5630, .T. ) ;
#9763=CIRCLE ( 'NONE', #6525, 6.000000000000005329 ) ;
#9768=ORIENTED_EDGE ( 'NONE', *, *, #22693, .F. ) ;
#9783=CARTESIAN_POINT ( 'NONE',  ( 167.4999999999996589, 494.4107529906318632, -84.99999999999995737 ) ) ;
#9808=CARTESIAN_POINT ( 'NONE',  ( 179.9999999999999147, -5.589247009368164321, 100.0000000000000142 ) ) ;
#9822=CARTESIAN_POINT ( 'NONE',  ( 179.9999999999999147, -5.589247009368136787, -84.99999999999997158 ) ) ;
#9849=DIRECTION ( 'NONE',  ( -1.000000000000000000, 2.696301922142074142E-31, -2.220446049250266932E-15 ) ) ;
#9899=FACE_OUTER_BOUND ( 'NONE', #11909, .T. ) ;
#9910=DIRECTION ( 'NONE',  ( -0.000000000000000000, -1.000000000000000000, -0.000000000000000000 ) ) ;
#9966=CARTESIAN_POINT ( 'NONE',  ( 167.4999999999996589, 494.4107529906318632, 84.99999999999995737 ) ) ;
#9994=AXIS2_PLACEMENT_3D ( 'NONE', #15334, #26501, #22602 ) ;
#10011=AXIS2_PLACEMENT_3D ( 'NONE', #1265, #14215, #23384 ) ;
#10016=VECTOR ( 'NONE', #17299, 1000.000000000000000 ) ;
#10042=ORIENTED_EDGE ( 'NONE', *, *, #6337, .T. ) ;
#10045=CARTESIAN_POINT ( 'NONE',  ( 179.9999999999999147, 526.4263741777961059, -84.99999999999997158 ) ) ;
#10114=ORIENTED_EDGE ( 'NONE', *, *, #7316, .T. ) ;
#10129=VECTOR ( 'NONE', #11708, 1000.000000000000000 ) ;
#10130=ORIENTED_EDGE ( 'NONE', *, *, #21243, .T. ) ;
#10166=ADVANCED_FACE ( 'NONE', ( #9235 ), #26321, .F. ) ;
#10167=VECTOR ( 'NONE', #19774, 1000.000000000000000 ) ;
#10208=VECTOR ( 'NONE', #9910, 1000.000000000000000 ) ;
#10232=DIRECTION ( 'NONE',  ( 2.220446049250266932E-15, -0.000000000000000000, 1.000000000000000000 ) ) ;
#10328=EDGE_CURVE ( 'NONE', #19372, #8066, #18459, .T. ) ;
#10358=AXIS2_PLACEMENT_3D ( 'NONE', #27360, #12445, #5958 ) ;
#10391=APPLICATION_CONTEXT ( 'automotive_design' ) ;
#10401=ORIENTED_EDGE ( 'NONE', *, *, #2599, .F. ) ;
#10431=( LENGTH_UNIT ( ) NAMED_UNIT ( * ) SI_UNIT ( .MILLI., .METRE. ) );
#10455=PLANE ( 'NONE',  #2677 ) ;
#10490=EDGE_CURVE ( 'NONE', #8066, #19372, #20743, .T. ) ;
#10492=CARTESIAN_POINT ( 'NONE',  ( 217.4999999999996305, -5.589247009368136787, -100.0000000000000142 ) ) ;
#10493=CARTESIAN_POINT ( 'NONE',  ( 187.4999999999996305, 133.0668745871126930, -36.86484227207694886 ) ) ;
#10543=ORIENTED_EDGE ( 'NONE', *, *, #14749, .F. ) ;
#10637=AXIS2_PLACEMENT_3D ( 'NONE', #25065, #2320, #14860 ) ;
#10729=LINE ( 'NONE', #8993, #15901 ) ;
#10808=EDGE_LOOP ( 'NONE', ( #12395, #2932, #12956, #7374 ) ) ;
#10817=EDGE_CURVE ( 'NONE', #24310, #25171, #9442, .T. ) ;
#10869=ORIENTED_EDGE ( 'NONE', *, *, #17914, .F. ) ;
#10870=FACE_OUTER_BOUND ( 'NONE', #8881, .T. ) ;
#10902=ORIENTED_EDGE ( 'NONE', *, *, #1018, .T. ) ;
#10906=LINE ( 'NONE', #4145, #9349 ) ;
#10911=DIRECTION ( 'NONE',  ( -0.000000000000000000, 1.000000000000000000, 1.214306433183764966E-16 ) ) ;
#10980=PLANE ( 'NONE',  #24067 ) ;
#10987=CARTESIAN_POINT ( 'NONE',  ( 167.4999999999996589, -5.589247009368157215, 84.99999999999995737 ) ) ;
#11000=CARTESIAN_POINT ( 'NONE',  ( 232.4999999999996305, 133.0668745871126930, 42.86484227207692044 ) ) ;
#11003=VECTOR ( 'NONE', #9035, 1000.000000000000000 ) ;
#11062=CARTESIAN_POINT ( 'NONE',  ( 217.4999999999996305, 494.4107529906318632, 100.0000000000000142 ) ) ;
#11063=ORIENTED_EDGE ( 'NONE', *, *, #8578, .T. ) ;
#11084=AXIS2_PLACEMENT_3D ( 'NONE', #27818, #28101, #21367 ) ;
#11099=VERTEX_POINT ( 'NONE', #1713 ) ;
#11110=CARTESIAN_POINT ( 'NONE',  ( 179.9999999999999147, 526.4263741777961059, 100.0000000000000142 ) ) ;
#11158=CARTESIAN_POINT ( 'NONE',  ( 217.4999999999996305, -5.589247009368160768, 100.0000000000000142 ) ) ;
#11249=( NAMED_UNIT ( * ) SI_UNIT ( $, .STERADIAN. ) SOLID_ANGLE_UNIT ( ) );
#11269=AXIS2_PLACEMENT_3D ( 'NONE', #8263, #17016, #25772 ) ;
#11372=DIRECTION ( 'NONE',  ( 0.000000000000000000, 0.000000000000000000, -1.000000000000000000 ) ) ;
#11379=ADVANCED_FACE ( 'NONE', ( #9899 ), #27396, .F. ) ;
#11386=PLANE ( 'NONE',  #21662 ) ;
#11457=DIRECTION ( 'NONE',  ( 1.000000000000000000, 0.000000000000000000, 0.000000000000000000 ) ) ;
#11558=VERTEX_POINT ( 'NONE', #24233 ) ;
#11679=FACE_OUTER_BOUND ( 'NONE', #9464, .T. ) ;
#11708=DIRECTION ( 'NONE',  ( 1.000000000000000000, 2.696301922142074142E-31, -2.220446049250266932E-15 ) ) ;
#11758=CARTESIAN_POINT ( 'NONE',  ( 232.4999999999996305, 83.06687458711267880, -36.86484227207694175 ) ) ;
#11765=PLANE ( 'NONE',  #24229 ) ;
#11819=ORIENTED_EDGE ( 'NONE', *, *, #8251, .F. ) ;
#11902=FACE_OUTER_BOUND ( 'NONE', #16969, .T. ) ;
#11909=EDGE_LOOP ( 'NONE', ( #5863, #15221, #27304, #16761 ) ) ;
#12015=CARTESIAN_POINT ( 'NONE',  ( 187.4999999999996305, 133.0668745871126930, -36.86484227207694886 ) ) ;
#12058=DIRECTION ( 'NONE',  ( 1.000000000000000000, 0.000000000000000000, 0.000000000000000000 ) ) ;
#12066=EDGE_CURVE ( 'NONE', #17060, #7044, #9355, .T. ) ;
#12073=AXIS2_PLACEMENT_3D ( 'NONE', #2867, #24421, #4730 ) ;
#12075=ORIENTED_EDGE ( 'NONE', *, *, #7614, .F. ) ;
#12089=FACE_BOUND ( 'NONE', #8511, .T. ) ;
#12138=ORIENTED_EDGE ( 'NONE', *, *, #10817, .T. ) ;
#12207=DIRECTION ( 'NONE',  ( 0.000000000000000000, 0.000000000000000000, -1.000000000000000000 ) ) ;
#12220=ORIENTED_EDGE ( 'NONE', *, *, #21007, .T. ) ;
#12303=DIRECTION ( 'NONE',  ( 1.000000000000000000, -0.000000000000000000, -0.000000000000000000 ) ) ;
#12320=AXIS2_PLACEMENT_3D ( 'NONE', #26987, #5154, #15661 ) ;
#12368=LINE ( 'NONE', #21106, #11003 ) ;
#12395=ORIENTED_EDGE ( 'NONE', *, *, #18802, .T. ) ;
#12439=DIRECTION ( 'NONE',  ( 0.000000000000000000, 0.000000000000000000, -1.000000000000000000 ) ) ;
#12445=DIRECTION ( 'NONE',  ( 1.000000000000000000, -0.000000000000000000, -0.000000000000000000 ) ) ;
#12485=PLANE ( 'NONE',  #11084 ) ;
#12562=DIRECTION ( 'NONE',  ( 0.000000000000000000, 0.000000000000000000, -1.000000000000000000 ) ) ;
#12703=CARTESIAN_POINT ( 'NONE',  ( 187.4999999999996305, 133.0668745871126930, 36.86484227207694886 ) ) ;
#12708=ORIENTED_EDGE ( 'NONE', *, *, #15165, .T. ) ;
#12719=PLANE ( 'NONE',  #27654 ) ;
#12772=LINE ( 'NONE', #23390, #6488 ) ;
#12836=EDGE_LOOP ( 'NONE', ( #25833, #8726 ) ) ;
#12869=LINE ( 'NONE', #8552, #10016 ) ;
#12885=ADVANCED_FACE ( 'NONE', ( #20212 ), #26961, .F. ) ;
#12942=EDGE_LOOP ( 'NONE', ( #11819, #21849, #23331, #17844 ) ) ;
#12956=ORIENTED_EDGE ( 'NONE', *, *, #15210, .T. ) ;
#13081=CARTESIAN_POINT ( 'NONE',  ( 167.4999999999996589, 494.4107529906318632, 74.99999999999995737 ) ) ;
#13106=EDGE_CURVE ( 'NONE', #15738, #27472, #22703, .T. ) ;
#13133=CIRCLE ( 'NONE', #23230, 5.999999999999991118 ) ;
#13136=CARTESIAN_POINT ( 'NONE',  ( 217.4999999999996305, 258.6181251126050711, 1.387778780781445676E-14 ) ) ;
#13156=DIRECTION ( 'NONE',  ( 1.000000000000000000, -0.000000000000000000, -0.000000000000000000 ) ) ;
#13178=ORIENTED_EDGE ( 'NONE', *, *, #18949, .T. ) ;
#13181=DIRECTION ( 'NONE',  ( 1.000000000000000000, -0.000000000000000000, -0.000000000000000000 ) ) ;
#13220=SHAPE_REPRESENTATION ( 'Sliding Carriage', ( #10637 ), #7887 ) ;
#13277=VERTEX_POINT ( 'NONE', #19747 ) ;
#13281=DIRECTION ( 'NONE',  ( 0.000000000000000000, 0.000000000000000000, -1.000000000000000000 ) ) ;
#13320=FACE_OUTER_BOUND ( 'NONE', #22558, .T. ) ;
#13327=FACE_OUTER_BOUND ( 'NONE', #20596, .T. ) ;
#13329=FACE_BOUND ( 'NONE', #23056, .T. ) ;
#13376=AXIS2_PLACEMENT_3D ( 'NONE', #19814, #17800, #13507 ) ;
#13452=ORIENTED_EDGE ( 'NONE', *, *, #28271, .T. ) ;
#13460=LINE ( 'NONE', #22069, #3866 ) ;
#13467=CARTESIAN_POINT ( 'NONE',  ( 217.4999999999996305, -5.589247009368136787, -100.0000000000000142 ) ) ;
#13470=ORIENTED_EDGE ( 'NONE', *, *, #19791, .F. ) ;
#13507=DIRECTION ( 'NONE',  ( 0.000000000000000000, 0.000000000000000000, -1.000000000000000000 ) ) ;
#13517=ORIENTED_EDGE ( 'NONE', *, *, #8300, .T. ) ;
#13550=( NAMED_UNIT ( * ) PLANE_ANGLE_UNIT ( ) SI_UNIT ( $, .RADIAN. ) );
#13679=DIRECTION ( 'NONE',  ( 0.000000000000000000, 0.000000000000000000, -1.000000000000000000 ) ) ;
#13759=DIRECTION ( 'NONE',  ( 0.000000000000000000, 0.000000000000000000, 1.000000000000000000 ) ) ;
#13778=AXIS2_PLACEMENT_3D ( 'NONE', #26960, #22517, #26823 ) ;
#13830=DIRECTION ( 'NONE',  ( 0.000000000000000000, 0.000000000000000000, -1.000000000000000000 ) ) ;
#13832=DIRECTION ( 'NONE',  ( 1.000000000000000000, 0.000000000000000000, 0.000000000000000000 ) ) ;
#13841=ORIENTED_EDGE ( 'NONE', *, *, #8120, .T. ) ;
#13932=EDGE_CURVE ( 'NONE', #8030, #4661, #1723, .T. ) ;
#14057=ORIENTED_EDGE ( 'NONE', *, *, #18084, .T. ) ;
#14167=ORIENTED_EDGE ( 'NONE', *, *, #8120, .F. ) ;
#14215=DIRECTION ( 'NONE',  ( 0.000000000000000000, 0.000000000000000000, 1.000000000000000000 ) ) ;
#14221=DIRECTION ( 'NONE',  ( 0.000000000000000000, 0.000000000000000000, 1.000000000000000000 ) ) ;
#14281=VERTEX_POINT ( 'NONE', #21001 ) ;
#14351=FACE_OUTER_BOUND ( 'NONE', #4242, .T. ) ;
#14396=AXIS2_PLACEMENT_3D ( 'NONE', #22185, #20024, #4932 ) ;
#14407=CARTESIAN_POINT ( 'NONE',  ( 217.4999999999996305, 258.6181251126050711, 6.025000000000016342 ) ) ;
#14447=EDGE_CURVE ( 'NONE', #4562, #24145, #9330, .T. ) ;
#14477=VERTEX_POINT ( 'NONE', #19950 ) ;
#14494=CARTESIAN_POINT ( 'NONE',  ( 217.4749999999996533, 258.6181251126050711, 6.000000000000019540 ) ) ;
#14518=EDGE_CURVE ( 'NONE', #18272, #18076, #13133, .T. ) ;
#14519=CARTESIAN_POINT ( 'NONE',  ( 187.4999999999996305, 0.000000000000000000, 0.000000000000000000 ) ) ;
#14549=CYLINDRICAL_SURFACE ( 'NONE', #3831, 5.999999999999977796 ) ;
#14559=ORIENTED_EDGE ( 'NONE', *, *, #15165, .F. ) ;
#14563=VERTEX_POINT ( 'NONE', #22827 ) ;
#14600=CARTESIAN_POINT ( 'NONE',  ( 217.4999999999996305, 133.0668745871126930, 36.86484227207694886 ) ) ;
#14688=DIRECTION ( 'NONE',  ( 0.000000000000000000, 0.000000000000000000, -1.000000000000000000 ) ) ;
#14749=EDGE_CURVE ( 'NONE', #27317, #21276, #15343, .T. ) ;
#14816=DIRECTION ( 'NONE',  ( 1.000000000000000000, -0.000000000000000000, -0.000000000000000000 ) ) ;
#14831=AXIS2_PLACEMENT_3D ( 'NONE', #4660, #8984, #80 ) ;
#14860=DIRECTION ( 'NONE',  ( 1.000000000000000000, 0.000000000000000000, 0.000000000000000000 ) ) ;
#14874=CARTESIAN_POINT ( 'NONE',  ( 179.9999999999999147, -5.589247009368138563, -84.99999999999997158 ) ) ;
#14897=CARTESIAN_POINT ( 'NONE',  ( 217.4999999999996305, 83.06687458711267880, 30.86484227207694886 ) ) ;
#14997=CARTESIAN_POINT ( 'NONE',  ( 217.4999999999996305, 494.4107529906318632, -100.0000000000000142 ) ) ;
#14998=ORIENTED_EDGE ( 'NONE', *, *, #19791, .T. ) ;
#15027=DIRECTION ( 'NONE',  ( 0.000000000000000000, 0.000000000000000000, -1.000000000000000000 ) ) ;
#15060=AXIS2_PLACEMENT_3D ( 'NONE', #21295, #7806, #3764 ) ;
#15094=CARTESIAN_POINT ( 'NONE',  ( 179.9999999999999147, -5.589247009368157215, 84.99999999999997158 ) ) ;
#15148=LINE ( 'NONE', #19724, #1988 ) ;
#15165=EDGE_CURVE ( 'NONE', #8650, #14563, #19738, .T. ) ;
#15200=FACE_OUTER_BOUND ( 'NONE', #16768, .T. ) ;
#15210=EDGE_CURVE ( 'NONE', #7037, #11558, #12869, .T. ) ;
#15212=ORIENTED_EDGE ( 'NONE', *, *, #4624, .F. ) ;
#15221=ORIENTED_EDGE ( 'NONE', *, *, #9683, .F. ) ;
#15240=DIRECTION ( 'NONE',  ( -1.000000000000000000, -0.000000000000000000, -0.000000000000000000 ) ) ;
#15243=ORIENTED_EDGE ( 'NONE', *, *, #7192, .T. ) ;
#15259=EDGE_LOOP ( 'NONE', ( #4524, #7689 ) ) ;
#15261=ORIENTED_EDGE ( 'NONE', *, *, #13932, .F. ) ;
#15334=CARTESIAN_POINT ( 'NONE',  ( 217.4999999999996305, 258.6181251126050711, 1.387778780781445676E-14 ) ) ;
#15343=LINE ( 'NONE', #28241, #3960 ) ;
#15346=FACE_BOUND ( 'NONE', #4377, .T. ) ;
#15420=EDGE_CURVE ( 'NONE', #24310, #27485, #7944, .T. ) ;
#15462=AXIS2_PLACEMENT_3D ( 'NONE', #22021, #2328, #6510 ) ;
#15481=DIRECTION ( 'NONE',  ( 0.000000000000000000, 0.000000000000000000, -1.000000000000000000 ) ) ;
#15496=ADVANCED_FACE ( 'NONE', ( #1194 ), #22848, .F. ) ;
#15510=UNCERTAINTY_MEASURE_WITH_UNIT (LENGTH_MEASURE( 1.000000000000000082E-05 ), #5050, 'distance_accuracy_value', 'NONE');
#15555=EDGE_CURVE ( 'NONE', #20391, #11099, #6776, .T. ) ;
#15616=AXIS2_PLACEMENT_3D ( 'NONE', #14519, #16946, #27841 ) ;
#15661=DIRECTION ( 'NONE',  ( 0.000000000000000000, 0.000000000000000000, -1.000000000000000000 ) ) ;
#15669=DIRECTION ( 'NONE',  ( -0.000000000000000000, 1.214306433183764720E-16, -1.000000000000000000 ) ) ;
#15695=CARTESIAN_POINT ( 'NONE',  ( 217.4999999999996305, 133.0668745871126930, 30.86484227207697018 ) ) ;
#15702=ADVANCED_FACE ( 'NONE', ( #11679 ), #17834, .F. ) ;
#15731=ORIENTED_EDGE ( 'NONE', *, *, #23804, .F. ) ;
#15738=VERTEX_POINT ( 'NONE', #15695 ) ;
#15765=EDGE_CURVE ( 'NONE', #27472, #15738, #23329, .T. ) ;
#15888=EDGE_CURVE ( 'NONE', #11099, #15738, #23992, .T. ) ;
#15901=VECTOR ( 'NONE', #20042, 1000.000000000000000 ) ;
#15913=CARTESIAN_POINT ( 'NONE',  ( 179.9999999999999147, 494.4107529906318632, -84.99999999999997158 ) ) ;
#15931=ORIENTED_EDGE ( 'NONE', *, *, #21007, .F. ) ;
#15984=DIRECTION ( 'NONE',  ( 1.000000000000000000, 0.000000000000000000, 0.000000000000000000 ) ) ;
#16000=ORIENTED_EDGE ( 'NONE', *, *, #25785, .T. ) ;
#16043=ADVANCED_FACE ( 'NONE', ( #19466 ), #8412, .F. ) ;
#16063=DIRECTION ( 'NONE',  ( 1.000000000000000000, -0.000000000000000000, -0.000000000000000000 ) ) ;
#16187=AXIS2_PLACEMENT_3D ( 'NONE', #10493, #27996, #17097 ) ;
#16288=AXIS2_PLACEMENT_3D ( 'NONE', #14600, #25644, #16479 ) ;
#16296=ORIENTED_EDGE ( 'NONE', *, *, #21218, .F. ) ;
#16300=CARTESIAN_POINT ( 'NONE',  ( 187.4999999999996305, 83.06687458711267880, -30.86484227207694886 ) ) ;
#16336=CARTESIAN_POINT ( 'NONE',  ( 167.4999999999996589, 494.4107529906318632, -74.99999999999995737 ) ) ;
#16357=ORIENTED_EDGE ( 'NONE', *, *, #19988, .T. ) ;
#16401=ADVANCED_BREP_SHAPE_REPRESENTATION ( '', ( #27970, #10637 ), #7887 ) ;
#16479=DIRECTION ( 'NONE',  ( 0.000000000000000000, 0.000000000000000000, -1.000000000000000000 ) ) ;
#16524=VERTEX_POINT ( 'NONE', #9966 ) ;
#16558=ORIENTED_EDGE ( 'NONE', *, *, #26274, .F. ) ;
#16577=VERTEX_POINT ( 'NONE', #26445 ) ;
#16664=ORIENTED_EDGE ( 'NONE', *, *, #14749, .T. ) ;
#16701=CARTESIAN_POINT ( 'NONE',  ( 179.9999999999999147, -5.589247009368136787, -100.0000000000000142 ) ) ;
#16761=ORIENTED_EDGE ( 'NONE', *, *, #4624, .T. ) ;
#16768=EDGE_LOOP ( 'NONE', ( #10902, #20509, #18332, #9768, #9448, #20564, #20890, #5733, #15731, #10401, #22119, #21102 ) ) ;
#16837=ORIENTED_EDGE ( 'NONE', *, *, #17041, .T. ) ;
#16870=DIRECTION ( 'NONE',  ( 1.000000000000000000, -0.000000000000000000, -0.000000000000000000 ) ) ;
#16879=CARTESIAN_POINT ( 'NONE',  ( 179.9999999999999147, -5.589247009368136787, -100.0000000000000142 ) ) ;
#16933=VERTEX_POINT ( 'NONE', #15094 ) ;
#16946=DIRECTION ( 'NONE',  ( 1.000000000000000000, 0.000000000000000000, 0.000000000000000000 ) ) ;
#16950=CARTESIAN_POINT ( 'NONE',  ( 187.4999999999996305, -5.589247009368140340, -74.99999999999995737 ) ) ;
#16969=EDGE_LOOP ( 'NONE', ( #16296, #19197, #20535, #4419 ) ) ;
#16973=CIRCLE ( 'NONE', #13778, 5.999999999999991118 ) ;
#17004=CARTESIAN_POINT ( 'NONE',  ( 217.4999999999996305, 258.6181251126050711, 1.387778780781445676E-14 ) ) ;
#17005=EDGE_LOOP ( 'NONE', ( #28141, #27699, #3393, #19937 ) ) ;
#17014=FACE_OUTER_BOUND ( 'NONE', #19516, .T. ) ;
#17016=DIRECTION ( 'NONE',  ( 1.000000000000000000, -0.000000000000000000, -0.000000000000000000 ) ) ;
#17041=EDGE_CURVE ( 'NONE', #14477, #4345, #18386, .T. ) ;
#17052=VECTOR ( 'NONE', #14221, 1000.000000000000000 ) ;
#17060=VERTEX_POINT ( 'NONE', #20049 ) ;
#17097=DIRECTION ( 'NONE',  ( 0.000000000000000000, 0.000000000000000000, -1.000000000000000000 ) ) ;
#17117=CARTESIAN_POINT ( 'NONE',  ( 179.9999999999999147, 526.4263741777961059, -84.99999999999997158 ) ) ;
#17158=LINE ( 'NONE', #16879, #20210 ) ;
#17163=ADVANCED_FACE ( 'NONE', ( #13320 ), #22070, .F. ) ;
#17202=FACE_OUTER_BOUND ( 'NONE', #10808, .T. ) ;
#17209=DIRECTION ( 'NONE',  ( 1.000000000000000000, -0.000000000000000000, -0.000000000000000000 ) ) ;
#17242=AXIS2_PLACEMENT_3D ( 'NONE', #130, #10911, #9040 ) ;
#17283=VECTOR ( 'NONE', #662, 1000.000000000000000 ) ;
#17299=DIRECTION ( 'NONE',  ( -0.000000000000000000, -1.000000000000000000, -0.000000000000000000 ) ) ;
#17383=PRODUCT_CONTEXT ( 'NONE', #3578, 'mechanical' ) ;
#17421=ADVANCED_FACE ( 'NONE', ( #17014 ), #27638, .F. ) ;
#17428=ORIENTED_EDGE ( 'NONE', *, *, #17914, .T. ) ;
#17452=LINE ( 'NONE', #6681, #22580 ) ;
#17501=DIRECTION ( 'NONE',  ( -0.000000000000000000, -1.000000000000000000, -0.000000000000000000 ) ) ;
#17565=ORIENTED_EDGE ( 'NONE', *, *, #6337, .F. ) ;
#17601=EDGE_CURVE ( 'NONE', #27317, #8030, #6878, .T. ) ;
#17691=DIRECTION ( 'NONE',  ( 0.000000000000000000, 0.000000000000000000, -1.000000000000000000 ) ) ;
#17800=DIRECTION ( 'NONE',  ( 1.000000000000000000, -0.000000000000000000, -0.000000000000000000 ) ) ;
#17834=PLANE ( 'NONE',  #19202 ) ;
#17844=ORIENTED_EDGE ( 'NONE', *, *, #18949, .F. ) ;
#17872=CARTESIAN_POINT ( 'NONE',  ( 232.4999999999996305, 83.06687458711267880, -42.86484227207692754 ) ) ;
#17897=AXIS2_PLACEMENT_3D ( 'NONE', #23206, #12303, #25770 ) ;
#17914=EDGE_CURVE ( 'NONE', #22044, #27664, #17158, .T. ) ;
#18026=AXIS2_PLACEMENT_3D ( 'NONE', #3672, #19050, #25933 ) ;
#18032=DIRECTION ( 'NONE',  ( -0.000000000000000000, -1.000000000000000000, -0.000000000000000000 ) ) ;
#18076=VERTEX_POINT ( 'NONE', #22890 ) ;
#18084=EDGE_CURVE ( 'NONE', #27485, #22044, #18441, .T. ) ;
#18092=EDGE_CURVE ( 'NONE', #9020, #7037, #5360, .T. ) ;
#18150=LINE ( 'NONE', #7654, #2855 ) ;
#18205=DIRECTION ( 'NONE',  ( -0.000000000000000000, -1.000000000000000000, -0.000000000000000000 ) ) ;
#18220=ADVANCED_FACE ( 'NONE', ( #27462 ), #3482, .F. ) ;
#18272=VERTEX_POINT ( 'NONE', #8081 ) ;
#18303=DIRECTION ( 'NONE',  ( 0.000000000000000000, 0.000000000000000000, 1.000000000000000000 ) ) ;
#18332=ORIENTED_EDGE ( 'NONE', *, *, #10817, .F. ) ;
#18386=LINE ( 'NONE', #9052, #19711 ) ;
#18393=EDGE_CURVE ( 'NONE', #18911, #24637, #6204, .T. ) ;
#18431=CIRCLE ( 'NONE', #18026, 5.999999999999991118 ) ;
#18441=LINE ( 'NONE', #9822, #10129 ) ;
#18452=VECTOR ( 'NONE', #13156, 1000.000000000000000 ) ;
#18459=CIRCLE ( 'NONE', #22576, 5.999999999999991118 ) ;
#18465=LINE ( 'NONE', #5100, #17283 ) ;
#18606=EDGE_LOOP ( 'NONE', ( #23713, #27177, #13517, #12220 ) ) ;
#18614=CYLINDRICAL_SURFACE ( 'NONE', #10358, 5.999999999999977796 ) ;
#18624=( NAMED_UNIT ( * ) SI_UNIT ( $, .STERADIAN. ) SOLID_ANGLE_UNIT ( ) );
#18636=EDGE_LOOP ( 'NONE', ( #28169, #16000, #10114, #10869 ) ) ;
#18673=ADVANCED_FACE ( 'NONE', ( #15200 ), #12485, .F. ) ;
#18710=CARTESIAN_POINT ( 'NONE',  ( 232.4999999999996305, 83.06687458711267880, 30.86484227207694886 ) ) ;
#18802=EDGE_CURVE ( 'NONE', #13277, #9020, #6568, .T. ) ;
#18815=CARTESIAN_POINT ( 'NONE',  ( 217.4999999999996305, 494.4107529906318632, 100.0000000000000142 ) ) ;
#18911=VERTEX_POINT ( 'NONE', #16336 ) ;
#18949=EDGE_CURVE ( 'NONE', #24145, #14477, #9445, .T. ) ;
#18987=ORIENTED_EDGE ( 'NONE', *, *, #831, .F. ) ;
#18999=DIRECTION ( 'NONE',  ( -1.000000000000000000, 0.000000000000000000, -2.220446049250266932E-15 ) ) ;
#19006=EDGE_LOOP ( 'NONE', ( #19009, #12138, #9170, #22733 ) ) ;
#19009=ORIENTED_EDGE ( 'NONE', *, *, #15420, .F. ) ;
#19046=DIRECTION ( 'NONE',  ( 0.7071067811865474617, 0.000000000000000000, -0.7071067811865474617 ) ) ;
#19050=DIRECTION ( 'NONE',  ( 1.000000000000000000, 0.000000000000000000, 0.000000000000000000 ) ) ;
#19154=EDGE_CURVE ( 'NONE', #11558, #13277, #22039, .T. ) ;
#19197=ORIENTED_EDGE ( 'NONE', *, *, #2599, .T. ) ;
#19202=AXIS2_PLACEMENT_3D ( 'NONE', #27020, #5041, #9075 ) ;
#19204=EDGE_CURVE ( 'NONE', #8066, #18076, #21763, .T. ) ;
#19216=CARTESIAN_POINT ( 'NONE',  ( 217.4999999999996305, 0.000000000000000000, 0.000000000000000000 ) ) ;
#19275=EDGE_CURVE ( 'NONE', #968, #9708, #21642, .T. ) ;
#19357=ORIENTED_EDGE ( 'NONE', *, *, #21902, .T. ) ;
#19372=VERTEX_POINT ( 'NONE', #16300 ) ;
#19378=CARTESIAN_POINT ( 'NONE',  ( 217.4999999999996305, 83.06687458711267880, 42.86484227207692754 ) ) ;
#19389=CARTESIAN_POINT ( 'NONE',  ( 232.4999999999996305, 133.0668745871126930, 30.86484227207697018 ) ) ;
#19445=ORIENTED_EDGE ( 'NONE', *, *, #1018, .F. ) ;
#19466=FACE_OUTER_BOUND ( 'NONE', #17005, .T. ) ;
#19516=EDGE_LOOP ( 'NONE', ( #4871, #20478, #26289, #22310 ) ) ;
#19706=DIRECTION ( 'NONE',  ( -1.000000000000000000, -0.000000000000000000, 0.000000000000000000 ) ) ;
#19711=VECTOR ( 'NONE', #15669, 1000.000000000000000 ) ;
#19724=CARTESIAN_POINT ( 'NONE',  ( 217.4999999999996305, -5.589247009368160768, 100.0000000000000142 ) ) ;
#19738=LINE ( 'NONE', #10987, #5876 ) ;
#19747=CARTESIAN_POINT ( 'NONE',  ( 217.4999999999996305, -5.589247009368136787, -100.0000000000000142 ) ) ;
#19749=DIRECTION ( 'NONE',  ( 1.000000000000000000, -0.000000000000000000, -0.000000000000000000 ) ) ;
#19774=DIRECTION ( 'NONE',  ( 0.000000000000000000, 1.000000000000000000, 0.000000000000000000 ) ) ;
#19791=EDGE_CURVE ( 'NONE', #8030, #27317, #9763, .T. ) ;
#19814=CARTESIAN_POINT ( 'NONE',  ( 217.4749999999996533, 258.6181251126050711, 1.387778780781445676E-14 ) ) ;
#19820=ADVANCED_FACE ( 'NONE', ( #20695 ), #11386, .F. ) ;
#19842=DIRECTION ( 'NONE',  ( -1.000000000000000000, 0.000000000000000000, -2.220446049250266932E-15 ) ) ;
#19866=DIRECTION ( 'NONE',  ( -1.000000000000000000, -0.000000000000000000, -0.000000000000000000 ) ) ;
#19873=CARTESIAN_POINT ( 'NONE',  ( 167.4999999999996589, 526.4263741777961059, 84.99999999999995737 ) ) ;
#19886=ORIENTED_EDGE ( 'NONE', *, *, #22919, .F. ) ;
#19911=DIRECTION ( 'NONE',  ( 0.000000000000000000, 0.000000000000000000, -1.000000000000000000 ) ) ;
#19928=EDGE_CURVE ( 'NONE', #22920, #2445, #24884, .T. ) ;
#19937=ORIENTED_EDGE ( 'NONE', *, *, #8300, .F. ) ;
#19950=CARTESIAN_POINT ( 'NONE',  ( 187.4999999999996305, -5.589247009368157215, 74.99999999999995737 ) ) ;
#19988=EDGE_CURVE ( 'NONE', #7037, #26389, #4581, .T. ) ;
#20003=ORIENTED_EDGE ( 'NONE', *, *, #15420, .T. ) ;
#20024=DIRECTION ( 'NONE',  ( 1.000000000000000000, 0.000000000000000000, 0.000000000000000000 ) ) ;
#20042=DIRECTION ( 'NONE',  ( 0.000000000000000000, 0.000000000000000000, -1.000000000000000000 ) ) ;
#20049=CARTESIAN_POINT ( 'NONE',  ( 217.4999999999996305, 133.0668745871126930, -30.86484227207697018 ) ) ;
#20135=CIRCLE ( 'NONE', #7761, 6.025000000000002132 ) ;
#20210=VECTOR ( 'NONE', #3655, 1000.000000000000000 ) ;
#20212=FACE_OUTER_BOUND ( 'NONE', #5977, .T. ) ;
#20220=ORIENTED_EDGE ( 'NONE', *, *, #1308, .T. ) ;
#20264=CARTESIAN_POINT ( 'NONE',  ( 217.4999999999996305, 258.6181251126050711, 1.387778780781445676E-14 ) ) ;
#20344=EDGE_CURVE ( 'NONE', #16524, #4562, #27402, .T. ) ;
#20381=CARTESIAN_POINT ( 'NONE',  ( 217.4999999999996305, 83.06687458711267880, -36.86484227207694175 ) ) ;
#20391=VERTEX_POINT ( 'NONE', #8415 ) ;
#20478=ORIENTED_EDGE ( 'NONE', *, *, #8847, .T. ) ;
#20490=PLANE ( 'NONE',  #26385 ) ;
#20509=ORIENTED_EDGE ( 'NONE', *, *, #25785, .F. ) ;
#20512=CARTESIAN_POINT ( 'NONE',  ( 187.4999999999996305, 258.6181251126050711, -5.999999999999991118 ) ) ;
#20535=ORIENTED_EDGE ( 'NONE', *, *, #831, .T. ) ;
#20564=ORIENTED_EDGE ( 'NONE', *, *, #8251, .T. ) ;
#20596=EDGE_LOOP ( 'NONE', ( #26785, #27278, #19445, #25100 ) ) ;
#20606=CARTESIAN_POINT ( 'NONE',  ( 167.4999999999996589, 526.4263741777961059, 74.99999999999995737 ) ) ;
#20695=FACE_OUTER_BOUND ( 'NONE', #27339, .T. ) ;
#20713=CARTESIAN_POINT ( 'NONE',  ( 217.4749999999996533, 258.6181251126050711, -5.999999999999991118 ) ) ;
#20743=CIRCLE ( 'NONE', #27176, 5.999999999999991118 ) ;
#20755=EDGE_CURVE ( 'NONE', #11099, #20391, #6120, .T. ) ;
#20759=DIRECTION ( 'NONE',  ( 1.000000000000000000, 0.000000000000000000, 0.000000000000000000 ) ) ;
#20799=AXIS2_PLACEMENT_3D ( 'NONE', #2302, #6907, #23 ) ;
#20810=PLANE ( 'NONE',  #10011 ) ;
#20851=CARTESIAN_POINT ( 'NONE',  ( 187.4999999999996305, 83.06687458711267880, -36.86484227207694175 ) ) ;
#20876=CIRCLE ( 'NONE', #6644, 5.999999999999977796 ) ;
#20890=ORIENTED_EDGE ( 'NONE', *, *, #14447, .F. ) ;
#20902=LINE ( 'NONE', #24939, #3791 ) ;
#20991=ORIENTED_EDGE ( 'NONE', *, *, #9177, .F. ) ;
#20997=ORIENTED_EDGE ( 'NONE', *, *, #20755, .T. ) ;
#21001=CARTESIAN_POINT ( 'NONE',  ( 187.4999999999996305, 83.06687458711267880, 30.86484227207694886 ) ) ;
#21003=DIRECTION ( 'NONE',  ( 2.220446049250266932E-15, 0.000000000000000000, -1.000000000000000000 ) ) ;
#21007=EDGE_CURVE ( 'NONE', #7044, #17060, #26307, .T. ) ;
#21032=ORIENTED_EDGE ( 'NONE', *, *, #22693, .T. ) ;
#21092=ORIENTED_EDGE ( 'NONE', *, *, #9177, .T. ) ;
#21102=ORIENTED_EDGE ( 'NONE', *, *, #18092, .F. ) ;
#21106=CARTESIAN_POINT ( 'NONE',  ( 217.4999999999996305, 494.4107529906318632, -100.0000000000000142 ) ) ;
#21123=ORIENTED_EDGE ( 'NONE', *, *, #8742, .F. ) ;
#21173=DIRECTION ( 'NONE',  ( 0.000000000000000000, 0.000000000000000000, -1.000000000000000000 ) ) ;
#21186=VECTOR ( 'NONE', #23918, 1000.000000000000000 ) ;
#21218=EDGE_CURVE ( 'NONE', #26389, #21355, #2330, .T. ) ;
#21243=EDGE_CURVE ( 'NONE', #11558, #21355, #15148, .T. ) ;
#21276=VERTEX_POINT ( 'NONE', #20713 ) ;
#21295=CARTESIAN_POINT ( 'NONE',  ( 217.4999999999996305, 258.6181251126050711, 1.387778780781445676E-14 ) ) ;
#21351=EDGE_CURVE ( 'NONE', #4661, #27627, #18150, .T. ) ;
#21354=VECTOR ( 'NONE', #14816, 1000.000000000000000 ) ;
#21355=VERTEX_POINT ( 'NONE', #9808 ) ;
#21367=DIRECTION ( 'NONE',  ( 0.000000000000000000, -0.000000000000000000, -1.000000000000000000 ) ) ;
#21369=VECTOR ( 'NONE', #22792, 1000.000000000000000 ) ;
#21457=CARTESIAN_POINT ( 'NONE',  ( 179.9999999999999147, 526.4263741777961059, -100.0000000000000142 ) ) ;
#21518=VERTEX_POINT ( 'NONE', #7306 ) ;
#21535=STYLED_ITEM('',(#28427),#27970);
#21545=LINE ( 'NONE', #10492, #5552 ) ;
#21556=AXIS2_PLACEMENT_3D ( 'NONE', #22214, #11457, #15481 ) ;
#21642=CIRCLE ( 'NONE', #25775, 5.999999999999991118 ) ;
#21662=AXIS2_PLACEMENT_3D ( 'NONE', #8050, #5612, #5889 ) ;
#21698=ORIENTED_EDGE ( 'NONE', *, *, #13932, .T. ) ;
#21763=LINE ( 'NONE', #17872, #18452 ) ;
#21803=DIRECTION ( 'NONE',  ( -0.000000000000000000, -1.000000000000000000, -0.000000000000000000 ) ) ;
#21849=ORIENTED_EDGE ( 'NONE', *, *, #2595, .T. ) ;
#21865=CARTESIAN_POINT ( 'NONE',  ( 167.4999999999996589, -5.589247009368136787, -74.99999999999995737 ) ) ;
#21902=EDGE_CURVE ( 'NONE', #16933, #8650, #20902, .T. ) ;
#21904=CONICAL_SURFACE ( 'NONE', #9994, 6.025000000000002132, 0.7853981633974482790 ) ;
#21960=DIRECTION ( 'NONE',  ( 1.000000000000000000, -0.000000000000000000, -0.000000000000000000 ) ) ;
#21977=PRODUCT_DEFINITION_SHAPE ( 'NONE', 'NONE',  #186 ) ;
#22021=CARTESIAN_POINT ( 'NONE',  ( 217.4999999999996305, 83.06687458711267880, -36.86484227207694175 ) ) ;
#22039=LINE ( 'NONE', #2345, #21186 ) ;
#22044=VERTEX_POINT ( 'NONE', #14874 ) ;
#22060=VECTOR ( 'NONE', #21803, 1000.000000000000000 ) ;
#22069=CARTESIAN_POINT ( 'NONE',  ( 232.4999999999996305, 83.06687458711267880, -30.86484227207694886 ) ) ;
#22070=PLANE ( 'NONE',  #26595 ) ;
#22099=ADVANCED_FACE ( 'NONE', ( #23479 ), #12719, .F. ) ;
#22119=ORIENTED_EDGE ( 'NONE', *, *, #19988, .F. ) ;
#22144=DIRECTION ( 'NONE',  ( 1.000000000000000000, 0.000000000000000000, 0.000000000000000000 ) ) ;
#22185=CARTESIAN_POINT ( 'NONE',  ( 217.4999999999996305, 133.0668745871126930, -36.86484227207694886 ) ) ;
#22214=CARTESIAN_POINT ( 'NONE',  ( 187.4999999999996305, 258.6181251126050711, 1.387778780781445676E-14 ) ) ;
#22241=ORIENTED_EDGE ( 'NONE', *, *, #1308, .F. ) ;
#22310=ORIENTED_EDGE ( 'NONE', *, *, #15888, .F. ) ;
#22428=ADVANCED_FACE ( 'NONE', ( #27595 ), #14549, .F. ) ;
#22446=DIRECTION ( 'NONE',  ( 1.000000000000000000, 0.000000000000000000, 0.000000000000000000 ) ) ;
#22510=DIRECTION ( 'NONE',  ( 1.000000000000000000, 0.000000000000000000, -0.000000000000000000 ) ) ;
#22517=DIRECTION ( 'NONE',  ( 1.000000000000000000, 0.000000000000000000, 0.000000000000000000 ) ) ;
#22536=ADVANCED_FACE ( 'NONE', ( #26160 ), #24160, .F. ) ;
#22557=ORIENTED_EDGE ( 'NONE', *, *, #18393, .T. ) ;
#22558=EDGE_LOOP ( 'NONE', ( #16357, #7965, #754, #6935 ) ) ;
#22576=AXIS2_PLACEMENT_3D ( 'NONE', #20851, #22446, #3039 ) ;
#22580=VECTOR ( 'NONE', #26212, 1000.000000000000000 ) ;
#22602=DIRECTION ( 'NONE',  ( 0.000000000000000000, 0.000000000000000000, -1.000000000000000000 ) ) ;
#22647=ORIENTED_EDGE ( 'NONE', *, *, #19275, .F. ) ;
#22688=DIRECTION ( 'NONE',  ( 0.000000000000000000, 0.000000000000000000, -1.000000000000000000 ) ) ;
#22693=EDGE_CURVE ( 'NONE', #18911, #24310, #24867, .T. ) ;
#22703=CIRCLE ( 'NONE', #16288, 5.999999999999977796 ) ;
#22733=ORIENTED_EDGE ( 'NONE', *, *, #18084, .F. ) ;
#22737=ORIENTED_EDGE ( 'NONE', *, *, #10490, .F. ) ;
#22782=ORIENTED_EDGE ( 'NONE', *, *, #21351, .F. ) ;
#22792=DIRECTION ( 'NONE',  ( 0.000000000000000000, 0.000000000000000000, -1.000000000000000000 ) ) ;
#22810=EDGE_LOOP ( 'NONE', ( #2207, #20991 ) ) ;
#22811=ORIENTED_EDGE ( 'NONE', *, *, #2140, .F. ) ;
#22827=CARTESIAN_POINT ( 'NONE',  ( 167.4999999999996589, -5.589247009368156327, 74.99999999999995737 ) ) ;
#22830=CARTESIAN_POINT ( 'NONE',  ( 167.4999999999996589, 494.4107529906318632, 74.99999999999995737 ) ) ;
#22848=CONICAL_SURFACE ( 'NONE', #15060, 6.025000000000002132, 0.7853981633974482790 ) ;
#22890=CARTESIAN_POINT ( 'NONE',  ( 217.4999999999996305, 83.06687458711267880, -42.86484227207692754 ) ) ;
#22919=EDGE_CURVE ( 'NONE', #16524, #8650, #10906, .T. ) ;
#22920=VERTEX_POINT ( 'NONE', #26542 ) ;
#22939=LINE ( 'NONE', #1240, #2821 ) ;
#22998=DIRECTION ( 'NONE',  ( 0.000000000000000000, 0.000000000000000000, -1.000000000000000000 ) ) ;
#23023=VECTOR ( 'NONE', #19749, 1000.000000000000000 ) ;
#23024=PLANE ( 'NONE',  #17242 ) ;
#23049=PRODUCT_DEFINITION_FORMATION_WITH_SPECIFIED_SOURCE ( 'ANY', '', #28144, .NOT_KNOWN. ) ;
#23056=EDGE_LOOP ( 'NONE', ( #23263, #25570 ) ) ;
#23174=CARTESIAN_POINT ( 'NONE',  ( 167.4999999999996589, 526.4263741777961059, -84.99999999999995737 ) ) ;
#23206=CARTESIAN_POINT ( 'NONE',  ( 232.4999999999996305, 133.0668745871126930, 36.86484227207694886 ) ) ;
#23230=AXIS2_PLACEMENT_3D ( 'NONE', #20381, #12058, #22688 ) ;
#23237=ORIENTED_EDGE ( 'NONE', *, *, #8847, .F. ) ;
#23263=ORIENTED_EDGE ( 'NONE', *, *, #13106, .F. ) ;
#23304=DIRECTION ( 'NONE',  ( 1.000000000000000000, -0.000000000000000000, -0.000000000000000000 ) ) ;
#23329=CIRCLE ( 'NONE', #23348, 5.999999999999977796 ) ;
#23331=ORIENTED_EDGE ( 'NONE', *, *, #17041, .F. ) ;
#23338=VECTOR ( 'NONE', #1543, 1000.000000000000000 ) ;
#23348=AXIS2_PLACEMENT_3D ( 'NONE', #607, #15984, #13830 ) ;
#23357=LINE ( 'NONE', #3669, #4676 ) ;
#23384=DIRECTION ( 'NONE',  ( 1.000000000000000000, 0.000000000000000000, -0.000000000000000000 ) ) ;
#23390=CARTESIAN_POINT ( 'NONE',  ( 232.4999999999996305, 133.0668745871126930, -42.86484227207692044 ) ) ;
#23426=ADVANCED_FACE ( 'NONE', ( #2195 ), #10980, .F. ) ;
#23429=VECTOR ( 'NONE', #19706, 1000.000000000000000 ) ;
#23479=FACE_OUTER_BOUND ( 'NONE', #18636, .T. ) ;
#23522=CARTESIAN_POINT ( 'NONE',  ( 187.4999999999996305, 133.0668745871126930, -30.86484227207697018 ) ) ;
#23578=ORIENTED_EDGE ( 'NONE', *, *, #20344, .T. ) ;
#23630=CYLINDRICAL_SURFACE ( 'NONE', #11269, 5.999999999999991118 ) ;
#23639=DIRECTION ( 'NONE',  ( 1.000000000000000000, -0.000000000000000000, -0.000000000000000000 ) ) ;
#23685=ORIENTED_EDGE ( 'NONE', *, *, #22919, .T. ) ;
#23710=CARTESIAN_POINT ( 'NONE',  ( 217.4999999999996305, 258.6181251126050711, 6.000000000000019540 ) ) ;
#23713=ORIENTED_EDGE ( 'NONE', *, *, #8845, .F. ) ;
#23804=EDGE_CURVE ( 'NONE', #3911, #16524, #2303, .T. ) ;
#23887=VECTOR ( 'NONE', #21960, 1000.000000000000000 ) ;
#23918=DIRECTION ( 'NONE',  ( -0.000000000000000000, 1.214306433183764720E-16, -1.000000000000000000 ) ) ;
#23992=LINE ( 'NONE', #19389, #2691 ) ;
#24067=AXIS2_PLACEMENT_3D ( 'NONE', #19873, #488, #13281 ) ;
#24132=CARTESIAN_POINT ( 'NONE',  ( 187.4999999999996305, 494.4107529906318632, 74.99999999999997158 ) ) ;
#24145=VERTEX_POINT ( 'NONE', #24132 ) ;
#24160=CYLINDRICAL_SURFACE ( 'NONE', #20799, 5.999999999999991118 ) ;
#24167=LINE ( 'NONE', #21865, #23429 ) ;
#24207=ORIENTED_EDGE ( 'NONE', *, *, #1373, .F. ) ;
#24224=CARTESIAN_POINT ( 'NONE',  ( 167.4999999999996589, -5.589247009368136787, -84.99999999999995737 ) ) ;
#24229=AXIS2_PLACEMENT_3D ( 'NONE', #24677, #7439, #1105 ) ;
#24232=FACE_BOUND ( 'NONE', #22810, .T. ) ;
#24233=CARTESIAN_POINT ( 'NONE',  ( 217.4999999999996305, -5.589247009368160768, 100.0000000000000142 ) ) ;
#24310=VERTEX_POINT ( 'NONE', #27127 ) ;
#24321=VECTOR ( 'NONE', #18303, 1000.000000000000000 ) ;
#24361=DIRECTION ( 'NONE',  ( -1.000000000000000000, 0.000000000000000000, -0.000000000000000000 ) ) ;
#24387=ORIENTED_EDGE ( 'NONE', *, *, #9752, .T. ) ;
#24421=DIRECTION ( 'NONE',  ( 1.000000000000000000, -0.000000000000000000, -0.000000000000000000 ) ) ;
#24454=DIRECTION ( 'NONE',  ( 1.000000000000000000, 0.000000000000000000, 0.000000000000000000 ) ) ;
#24462=DIRECTION ( 'NONE',  ( 0.000000000000000000, 0.000000000000000000, -1.000000000000000000 ) ) ;
#24610=ADVANCED_FACE ( 'NONE', ( #13327 ), #20490, .F. ) ;
#24637=VERTEX_POINT ( 'NONE', #531 ) ;
#24677=CARTESIAN_POINT ( 'NONE',  ( 179.9999999999999147, 526.4263741777961059, 100.0000000000000142 ) ) ;
#24756=DIRECTION ( 'NONE',  ( 0.7071067811865474617, 8.659560562354932858E-17, 0.7071067811865474617 ) ) ;
#24827=EDGE_LOOP ( 'NONE', ( #15931, #27109 ) ) ;
#24867=LINE ( 'NONE', #9783, #26304 ) ;
#24884=CIRCLE ( 'NONE', #16187, 5.999999999999977796 ) ;
#24900=ORIENTED_EDGE ( 'NONE', *, *, #3548, .T. ) ;
#24934=AXIS2_PLACEMENT_3D ( 'NONE', #12703, #3773, #12562 ) ;
#24939=CARTESIAN_POINT ( 'NONE',  ( 179.9999999999999147, -5.589247009368157215, 84.99999999999997158 ) ) ;
#25041=ORIENTED_EDGE ( 'NONE', *, *, #674, .T. ) ;
#25065=CARTESIAN_POINT ( 'NONE',  ( 0.000000000000000000, 0.000000000000000000, 0.000000000000000000 ) ) ;
#25100=ORIENTED_EDGE ( 'NONE', *, *, #18802, .F. ) ;
#25171=VERTEX_POINT ( 'NONE', #3643 ) ;
#25279=LINE ( 'NONE', #3018, #4545 ) ;
#25465=VECTOR ( 'NONE', #4529, 1000.000000000000000 ) ;
#25570=ORIENTED_EDGE ( 'NONE', *, *, #15765, .F. ) ;
#25615=ORIENTED_EDGE ( 'NONE', *, *, #26008, .T. ) ;
#25644=DIRECTION ( 'NONE',  ( 1.000000000000000000, 0.000000000000000000, 0.000000000000000000 ) ) ;
#25727=DIRECTION ( 'NONE',  ( 1.000000000000000000, 0.000000000000000000, -2.220446049250266932E-15 ) ) ;
#25732=VECTOR ( 'NONE', #4184, 1000.000000000000000 ) ;
#25770=DIRECTION ( 'NONE',  ( 0.000000000000000000, 0.000000000000000000, -1.000000000000000000 ) ) ;
#25772=DIRECTION ( 'NONE',  ( 0.000000000000000000, 0.000000000000000000, -1.000000000000000000 ) ) ;
#25775=AXIS2_PLACEMENT_3D ( 'NONE', #4499, #6671, #209 ) ;
#25785=EDGE_CURVE ( 'NONE', #25171, #6014, #10729, .T. ) ;
#25833=ORIENTED_EDGE ( 'NONE', *, *, #19928, .T. ) ;
#25837=ORIENTED_EDGE ( 'NONE', *, *, #19275, .T. ) ;
#25933=DIRECTION ( 'NONE',  ( 0.000000000000000000, 0.000000000000000000, -1.000000000000000000 ) ) ;
#25969=VECTOR ( 'NONE', #2560, 1000.000000000000000 ) ;
#26008=EDGE_CURVE ( 'NONE', #21355, #16933, #18465, .T. ) ;
#26010=PLANE ( 'NONE',  #2703 ) ;
#26011=EDGE_LOOP ( 'NONE', ( #15261, #4443, #16664, #24387 ) ) ;
#26047=ADVANCED_FACE ( 'NONE', ( #6087 ), #8247, .F. ) ;
#26160=FACE_OUTER_BOUND ( 'NONE', #27220, .T. ) ;
#26212=DIRECTION ( 'NONE',  ( 1.000000000000000000, -0.000000000000000000, -0.000000000000000000 ) ) ;
#26274=EDGE_CURVE ( 'NONE', #18076, #18272, #6723, .T. ) ;
#26289=ORIENTED_EDGE ( 'NONE', *, *, #15765, .T. ) ;
#26304=VECTOR ( 'NONE', #13679, 1000.000000000000000 ) ;
#26307=CIRCLE ( 'NONE', #26769, 5.999999999999977796 ) ;
#26320=ORIENTED_EDGE ( 'NONE', *, *, #8742, .T. ) ;
#26321=CYLINDRICAL_SURFACE ( 'NONE', #26680, 6.000000000000005329 ) ;
#26379=LINE ( 'NONE', #4270, #22060 ) ;
#26385=AXIS2_PLACEMENT_3D ( 'NONE', #5115, #13759, #22510 ) ;
#26389=VERTEX_POINT ( 'NONE', #7229 ) ;
#26415=CARTESIAN_POINT ( 'NONE',  ( 187.4999999999996305, 83.06687458711267880, -42.86484227207692754 ) ) ;
#26445=CARTESIAN_POINT ( 'NONE',  ( 187.4999999999996305, 494.4107529906318632, -74.99999999999995737 ) ) ;
#26501=DIRECTION ( 'NONE',  ( 1.000000000000000000, -0.000000000000000000, -0.000000000000000000 ) ) ;
#26542=CARTESIAN_POINT ( 'NONE',  ( 187.4999999999996305, 133.0668745871126930, -42.86484227207692044 ) ) ;
#26595=AXIS2_PLACEMENT_3D ( 'NONE', #11158, #19911, #24361 ) ;
#26674=EDGE_LOOP ( 'NONE', ( #10130, #25615, #19357, #12708, #24900, #16837, #434, #2014, #14057, #17428, #9690, #3670 ) ) ;
#26680=AXIS2_PLACEMENT_3D ( 'NONE', #13136, #2183, #24462 ) ;
#26682=VECTOR ( 'NONE', #18032, 1000.000000000000000 ) ;
#26769=AXIS2_PLACEMENT_3D ( 'NONE', #181, #24454, #4763 ) ;
#26785=ORIENTED_EDGE ( 'NONE', *, *, #7994, .T. ) ;
#26808=DIRECTION ( 'NONE',  ( 0.000000000000000000, 0.000000000000000000, -1.000000000000000000 ) ) ;
#26823=DIRECTION ( 'NONE',  ( 0.000000000000000000, 0.000000000000000000, -1.000000000000000000 ) ) ;
#26876=DIRECTION ( 'NONE',  ( 1.000000000000000000, -0.000000000000000000, -0.000000000000000000 ) ) ;
#26927=ORIENTED_EDGE ( 'NONE', *, *, #28271, .F. ) ;
#26960=CARTESIAN_POINT ( 'NONE',  ( 187.4999999999996305, 83.06687458711267880, 36.86484227207694175 ) ) ;
#26961=CYLINDRICAL_SURFACE ( 'NONE', #2962, 5.999999999999991118 ) ;
#26987=CARTESIAN_POINT ( 'NONE',  ( 217.4999999999996305, 83.06687458711267880, 36.86484227207694175 ) ) ;
#26991=CARTESIAN_POINT ( 'NONE',  ( 187.4999999999996305, 494.4107529906318632, -100.0000000000000142 ) ) ;
#27020=CARTESIAN_POINT ( 'NONE',  ( 167.4999999999996589, 526.4263741777961059, -84.99999999999995737 ) ) ;
#27090=CARTESIAN_POINT ( 'NONE',  ( 179.9999999999999147, 494.4107529906318632, 100.0000000000000142 ) ) ;
#27109=ORIENTED_EDGE ( 'NONE', *, *, #12066, .F. ) ;
#27127=CARTESIAN_POINT ( 'NONE',  ( 167.4999999999996589, 494.4107529906318632, -84.99999999999995737 ) ) ;
#27172=VECTOR ( 'NONE', #15240, 1000.000000000000000 ) ;
#27176=AXIS2_PLACEMENT_3D ( 'NONE', #9058, #2291, #156 ) ;
#27177=ORIENTED_EDGE ( 'NONE', *, *, #19928, .F. ) ;
#27193=CARTESIAN_POINT ( 'NONE',  ( 217.4999999999996305, 494.4107529906318632, -100.0000000000000142 ) ) ;
#27220=EDGE_LOOP ( 'NONE', ( #8810, #20220, #9596, #444 ) ) ;
#27272=VECTOR ( 'NONE', #19842, 1000.000000000000000 ) ;
#27278=ORIENTED_EDGE ( 'NONE', *, *, #7316, .F. ) ;
#27304=ORIENTED_EDGE ( 'NONE', *, *, #2140, .T. ) ;
#27317=VERTEX_POINT ( 'NONE', #20512 ) ;
#27339=EDGE_LOOP ( 'NONE', ( #1831, #11063, #22557, #12075 ) ) ;
#27360=CARTESIAN_POINT ( 'NONE',  ( 232.4999999999996305, 133.0668745871126930, -36.86484227207694886 ) ) ;
#27363=CARTESIAN_POINT ( 'NONE',  ( 187.4999999999996305, 526.4263741777961059, 74.99999999999995737 ) ) ;
#27396=CYLINDRICAL_SURFACE ( 'NONE', #159, 5.999999999999991118 ) ;
#27402=LINE ( 'NONE', #4092, #3793 ) ;
#27418=VECTOR ( 'NONE', #3485, 1000.000000000000000 ) ;
#27427=MECHANICAL_DESIGN_GEOMETRIC_PRESENTATION_REPRESENTATION('',(#21535),#6861);
#27462=FACE_OUTER_BOUND ( 'NONE', #28079, .T. ) ;
#27472=VERTEX_POINT ( 'NONE', #9533 ) ;
#27485=VERTEX_POINT ( 'NONE', #9393 ) ;
#27595=FACE_OUTER_BOUND ( 'NONE', #76, .T. ) ;
#27627=VERTEX_POINT ( 'NONE', #14407 ) ;
#27638=CYLINDRICAL_SURFACE ( 'NONE', #17897, 5.999999999999977796 ) ;
#27654=AXIS2_PLACEMENT_3D ( 'NONE', #21457, #1774, #12439 ) ;
#27664=VERTEX_POINT ( 'NONE', #16701 ) ;
#27672=CARTESIAN_POINT ( 'NONE',  ( 167.4999999999996589, -5.589247009368157215, 74.99999999999995737 ) ) ;
#27690=ORIENTED_EDGE ( 'NONE', *, *, #21902, .F. ) ;
#27699=ORIENTED_EDGE ( 'NONE', *, *, #8845, .T. ) ;
#27799=ORIENTED_EDGE ( 'NONE', *, *, #9683, .T. ) ;
#27818=CARTESIAN_POINT ( 'NONE',  ( 217.4999999999996305, 494.4107529906318632, -100.0000000000000142 ) ) ;
#27841=DIRECTION ( 'NONE',  ( 0.000000000000000000, 0.000000000000000000, -1.000000000000000000 ) ) ;
#27858=SHAPE_DEFINITION_REPRESENTATION ( #21977, #13220 ) ;
#27874=ADVANCED_FACE ( 'NONE', ( #11902 ), #11765, .F. ) ;
#27915=FACE_OUTER_BOUND ( 'NONE', #447, .T. ) ;
#27958=DIRECTION ( 'NONE',  ( 1.000000000000000000, 0.000000000000000000, 0.000000000000000000 ) ) ;
#27970=MANIFOLD_SOLID_BREP ( '\X2\00d8\X0\12.0mm Dowel Hole3[2]', #3996 ) ;
#27996=DIRECTION ( 'NONE',  ( 1.000000000000000000, 0.000000000000000000, 0.000000000000000000 ) ) ;
#28079=EDGE_LOOP ( 'NONE', ( #18987, #2152, #23685, #27690 ) ) ;
#28101=DIRECTION ( 'NONE',  ( 0.000000000000000000, -1.000000000000000000, 0.000000000000000000 ) ) ;
#28141=ORIENTED_EDGE ( 'NONE', *, *, #1540, .F. ) ;
#28144=PRODUCT ( 'Sliding Carriage', 'Sliding Carriage', '', ( #17383 ) ) ;
#28169=ORIENTED_EDGE ( 'NONE', *, *, #9262, .F. ) ;
#28241=CARTESIAN_POINT ( 'NONE',  ( 217.4999999999996305, 258.6181251126050711, -5.999999999999991118 ) ) ;
#28271=EDGE_CURVE ( 'NONE', #4562, #14563, #9418, .T. ) ;
#28392=ORIENTED_EDGE ( 'NONE', *, *, #3548, .F. ) ;
#28421=COLOUR_RGB('Light Blue',0.38,0.62,0.78);
#28422=FILL_AREA_STYLE_COLOUR('',#28421);
#28423=FILL_AREA_STYLE('',(#28422));
#28424=SURFACE_STYLE_FILL_AREA(#28423);
#28425=SURFACE_SIDE_STYLE('',(#28424));
#28426=SURFACE_STYLE_USAGE(.BOTH.,#28425);
#28427=PRESENTATION_STYLE_ASSIGNMENT((#28426));
ENDSEC;
END-ISO-10303-21;
